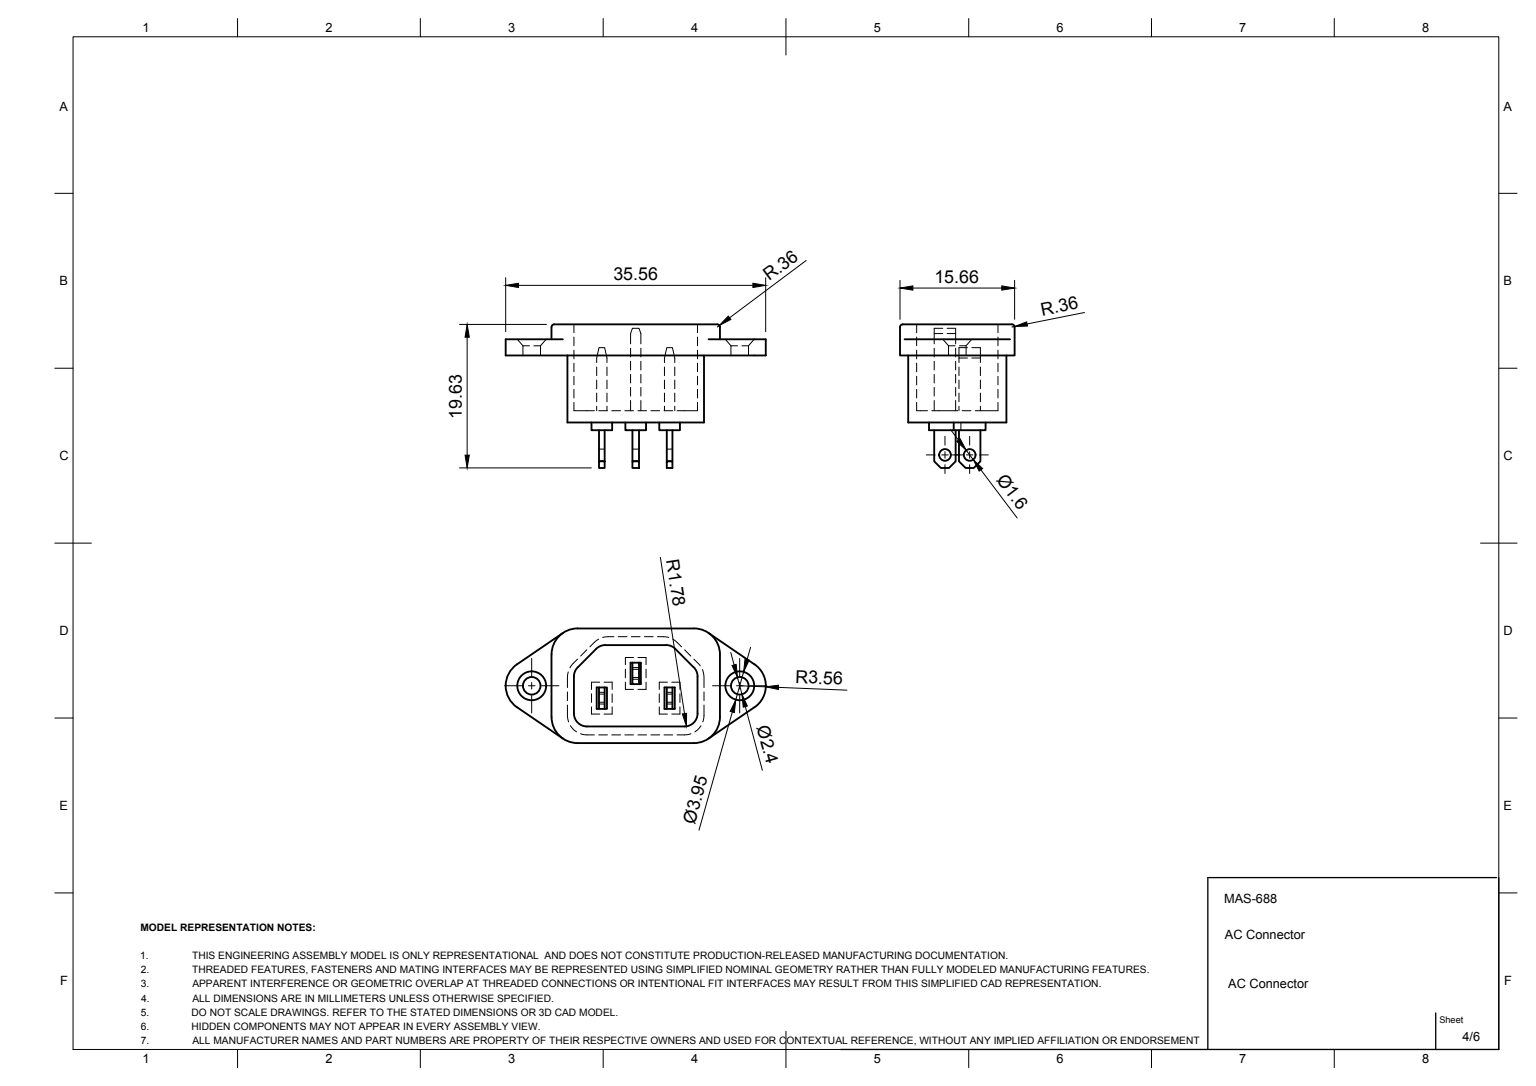
ISO-10303-21;
HEADER;
/* Generated by software containing ST-Developer
 * from STEP Tools, Inc. (www.steptools.com) 
 */

FILE_DESCRIPTION(
/* description */ ('STEP AP214'),
/* implementation_level */ '2;1');

FILE_NAME(
/* name */ 'AC Connector.step',
/* time_stamp */ '2026-11-14T03:58:36-08:00',
/* author */ (''),
/* organization */ (''),
/* preprocessor_version */ 'ST-DEVELOPER v20.2',
/* originating_system */ 'Autodesk Translation Framework v15.17.0.0',
/* authorisation */ '');

FILE_SCHEMA (('AUTOMOTIVE_DESIGN { 1 0 10303 214 3 1 1 }'));
ENDSEC;

DATA;
#10=MECHANICAL_DESIGN_GEOMETRIC_PRESENTATION_REPRESENTATION('',(#42),#65304);
#31=CONICAL_SURFACE('',#41051,1.97294590991864,0.71558499331768);
#32=CONICAL_SURFACE('',#41055,1.97294590991864,0.71558499331768);
#34=SHAPE_REPRESENTATION_RELATIONSHIP('SRR','None',#65325,#38);
#38=ADVANCED_BREP_SHAPE_REPRESENTATION('',(#46),#65301);
#42=STYLED_ITEM('',(#65354),#46);
#46=MANIFOLD_SOLID_BREP('Body1',#39934);
#226=FACE_BOUND('',#4996,.T.);
#227=FACE_BOUND('',#4997,.T.);
#228=FACE_BOUND('',#4998,.T.);
#229=FACE_BOUND('',#5012,.T.);
#230=FACE_BOUND('',#5013,.T.);
#231=FACE_BOUND('',#5014,.T.);
#232=FACE_BOUND('',#5016,.T.);
#233=FACE_BOUND('',#5018,.T.);
#234=FACE_BOUND('',#5019,.T.);
#235=FACE_BOUND('',#5020,.T.);
#236=FACE_BOUND('',#5033,.T.);
#237=FACE_BOUND('',#5037,.T.);
#238=FACE_BOUND('',#5080,.T.);
#239=FACE_BOUND('',#5090,.T.);
#240=FACE_BOUND('',#5093,.T.);
#241=FACE_BOUND('',#5099,.T.);
#242=FACE_BOUND('',#5106,.T.);
#243=FACE_BOUND('',#5108,.T.);
#244=FACE_BOUND('',#5110,.T.);
#245=FACE_BOUND('',#5121,.T.);
#246=FACE_BOUND('',#5123,.T.);
#887=PLANE('',#41066);
#888=PLANE('',#41073);
#889=PLANE('',#41074);
#890=PLANE('',#41075);
#891=PLANE('',#41076);
#892=PLANE('',#41077);
#893=PLANE('',#41078);
#894=PLANE('',#41079);
#895=PLANE('',#41080);
#896=PLANE('',#41081);
#897=PLANE('',#41082);
#898=PLANE('',#41083);
#899=PLANE('',#41084);
#900=PLANE('',#41085);
#901=PLANE('',#41092);
#902=PLANE('',#41103);
#903=PLANE('',#41118);
#904=PLANE('',#41122);
#905=PLANE('',#41126);
#906=PLANE('',#41130);
#907=PLANE('',#41131);
#908=PLANE('',#41134);
#909=PLANE('',#41135);
#910=PLANE('',#41136);
#911=PLANE('',#41137);
#912=PLANE('',#41138);
#913=PLANE('',#41156);
#914=PLANE('',#41158);
#915=PLANE('',#41160);
#916=PLANE('',#41162);
#917=PLANE('',#41164);
#918=PLANE('',#41166);
#919=PLANE('',#41168);
#920=PLANE('',#41170);
#921=PLANE('',#41172);
#922=PLANE('',#41174);
#923=PLANE('',#41176);
#924=PLANE('',#41178);
#925=PLANE('',#41179);
#926=PLANE('',#41180);
#927=PLANE('',#41181);
#928=PLANE('',#41182);
#929=PLANE('',#41183);
#930=PLANE('',#41184);
#931=PLANE('',#41185);
#932=PLANE('',#41186);
#933=PLANE('',#41187);
#934=PLANE('',#41188);
#935=PLANE('',#41189);
#936=PLANE('',#41190);
#937=PLANE('',#41191);
#938=PLANE('',#41192);
#939=PLANE('',#41193);
#940=PLANE('',#41194);
#941=PLANE('',#41195);
#942=PLANE('',#41196);
#943=PLANE('',#41197);
#944=PLANE('',#41198);
#945=PLANE('',#41199);
#946=PLANE('',#41200);
#947=PLANE('',#41201);
#948=PLANE('',#41202);
#949=PLANE('',#41203);
#950=PLANE('',#41204);
#951=PLANE('',#41205);
#952=PLANE('',#41206);
#953=PLANE('',#41207);
#954=PLANE('',#41208);
#955=PLANE('',#41209);
#956=PLANE('',#41210);
#957=PLANE('',#41211);
#958=PLANE('',#41212);
#959=PLANE('',#41213);
#960=PLANE('',#41214);
#961=PLANE('',#41215);
#962=PLANE('',#41216);
#963=PLANE('',#41217);
#964=PLANE('',#41218);
#965=PLANE('',#41219);
#966=PLANE('',#41220);
#967=PLANE('',#41221);
#968=PLANE('',#41222);
#969=PLANE('',#41223);
#2185=TOROIDAL_SURFACE('',#41139,3.2004,0.3556);
#2186=TOROIDAL_SURFACE('',#41146,3.2004,0.3556);
#2187=TOROIDAL_SURFACE('',#41148,3.2004,0.3556);
#2188=TOROIDAL_SURFACE('',#41154,3.2004,0.3556);
#2895=FACE_OUTER_BOUND('',#4987,.T.);
#2896=FACE_OUTER_BOUND('',#4988,.T.);
#2897=FACE_OUTER_BOUND('',#4989,.T.);
#2898=FACE_OUTER_BOUND('',#4990,.T.);
#2899=FACE_OUTER_BOUND('',#4991,.T.);
#2900=FACE_OUTER_BOUND('',#4992,.T.);
#2901=FACE_OUTER_BOUND('',#4993,.T.);
#2902=FACE_OUTER_BOUND('',#4994,.T.);
#2903=FACE_OUTER_BOUND('',#4995,.T.);
#2904=FACE_OUTER_BOUND('',#4999,.T.);
#2905=FACE_OUTER_BOUND('',#5000,.T.);
#2906=FACE_OUTER_BOUND('',#5001,.T.);
#2907=FACE_OUTER_BOUND('',#5002,.T.);
#2908=FACE_OUTER_BOUND('',#5003,.T.);
#2909=FACE_OUTER_BOUND('',#5004,.T.);
#2910=FACE_OUTER_BOUND('',#5005,.T.);
#2911=FACE_OUTER_BOUND('',#5006,.T.);
#2912=FACE_OUTER_BOUND('',#5007,.T.);
#2913=FACE_OUTER_BOUND('',#5008,.T.);
#2914=FACE_OUTER_BOUND('',#5009,.T.);
#2915=FACE_OUTER_BOUND('',#5010,.T.);
#2916=FACE_OUTER_BOUND('',#5011,.T.);
#2917=FACE_OUTER_BOUND('',#5015,.T.);
#2918=FACE_OUTER_BOUND('',#5017,.T.);
#2919=FACE_OUTER_BOUND('',#5021,.T.);
#2920=FACE_OUTER_BOUND('',#5022,.T.);
#2921=FACE_OUTER_BOUND('',#5023,.T.);
#2922=FACE_OUTER_BOUND('',#5024,.T.);
#2923=FACE_OUTER_BOUND('',#5025,.T.);
#2924=FACE_OUTER_BOUND('',#5026,.T.);
#2925=FACE_OUTER_BOUND('',#5027,.T.);
#2926=FACE_OUTER_BOUND('',#5028,.T.);
#2927=FACE_OUTER_BOUND('',#5029,.T.);
#2928=FACE_OUTER_BOUND('',#5030,.T.);
#2929=FACE_OUTER_BOUND('',#5031,.T.);
#2930=FACE_OUTER_BOUND('',#5032,.T.);
#2931=FACE_OUTER_BOUND('',#5034,.T.);
#2932=FACE_OUTER_BOUND('',#5035,.T.);
#2933=FACE_OUTER_BOUND('',#5036,.T.);
#2934=FACE_OUTER_BOUND('',#5038,.T.);
#2935=FACE_OUTER_BOUND('',#5039,.T.);
#2936=FACE_OUTER_BOUND('',#5040,.T.);
#2937=FACE_OUTER_BOUND('',#5041,.T.);
#2938=FACE_OUTER_BOUND('',#5042,.T.);
#2939=FACE_OUTER_BOUND('',#5043,.T.);
#2940=FACE_OUTER_BOUND('',#5044,.T.);
#2941=FACE_OUTER_BOUND('',#5045,.T.);
#2942=FACE_OUTER_BOUND('',#5046,.T.);
#2943=FACE_OUTER_BOUND('',#5047,.T.);
#2944=FACE_OUTER_BOUND('',#5048,.T.);
#2945=FACE_OUTER_BOUND('',#5049,.T.);
#2946=FACE_OUTER_BOUND('',#5050,.T.);
#2947=FACE_OUTER_BOUND('',#5051,.T.);
#2948=FACE_OUTER_BOUND('',#5052,.T.);
#2949=FACE_OUTER_BOUND('',#5053,.T.);
#2950=FACE_OUTER_BOUND('',#5054,.T.);
#2951=FACE_OUTER_BOUND('',#5055,.T.);
#2952=FACE_OUTER_BOUND('',#5056,.T.);
#2953=FACE_OUTER_BOUND('',#5057,.T.);
#2954=FACE_OUTER_BOUND('',#5058,.T.);
#2955=FACE_OUTER_BOUND('',#5059,.T.);
#2956=FACE_OUTER_BOUND('',#5060,.T.);
#2957=FACE_OUTER_BOUND('',#5061,.T.);
#2958=FACE_OUTER_BOUND('',#5062,.T.);
#2959=FACE_OUTER_BOUND('',#5063,.T.);
#2960=FACE_OUTER_BOUND('',#5064,.T.);
#2961=FACE_OUTER_BOUND('',#5065,.T.);
#2962=FACE_OUTER_BOUND('',#5066,.T.);
#2963=FACE_OUTER_BOUND('',#5067,.T.);
#2964=FACE_OUTER_BOUND('',#5068,.T.);
#2965=FACE_OUTER_BOUND('',#5069,.T.);
#2966=FACE_OUTER_BOUND('',#5070,.T.);
#2967=FACE_OUTER_BOUND('',#5071,.T.);
#2968=FACE_OUTER_BOUND('',#5072,.T.);
#2969=FACE_OUTER_BOUND('',#5073,.T.);
#2970=FACE_OUTER_BOUND('',#5074,.T.);
#2971=FACE_OUTER_BOUND('',#5075,.T.);
#2972=FACE_OUTER_BOUND('',#5076,.T.);
#2973=FACE_OUTER_BOUND('',#5077,.T.);
#2974=FACE_OUTER_BOUND('',#5078,.T.);
#2975=FACE_OUTER_BOUND('',#5079,.T.);
#2976=FACE_OUTER_BOUND('',#5081,.T.);
#2977=FACE_OUTER_BOUND('',#5082,.T.);
#2978=FACE_OUTER_BOUND('',#5083,.T.);
#2979=FACE_OUTER_BOUND('',#5084,.T.);
#2980=FACE_OUTER_BOUND('',#5085,.T.);
#2981=FACE_OUTER_BOUND('',#5086,.T.);
#2982=FACE_OUTER_BOUND('',#5087,.T.);
#2983=FACE_OUTER_BOUND('',#5088,.T.);
#2984=FACE_OUTER_BOUND('',#5089,.T.);
#2985=FACE_OUTER_BOUND('',#5091,.T.);
#2986=FACE_OUTER_BOUND('',#5092,.T.);
#2987=FACE_OUTER_BOUND('',#5094,.T.);
#2988=FACE_OUTER_BOUND('',#5095,.T.);
#2989=FACE_OUTER_BOUND('',#5096,.T.);
#2990=FACE_OUTER_BOUND('',#5097,.T.);
#2991=FACE_OUTER_BOUND('',#5098,.T.);
#2992=FACE_OUTER_BOUND('',#5100,.T.);
#2993=FACE_OUTER_BOUND('',#5101,.T.);
#2994=FACE_OUTER_BOUND('',#5102,.T.);
#2995=FACE_OUTER_BOUND('',#5103,.T.);
#2996=FACE_OUTER_BOUND('',#5104,.T.);
#2997=FACE_OUTER_BOUND('',#5105,.T.);
#2998=FACE_OUTER_BOUND('',#5107,.T.);
#2999=FACE_OUTER_BOUND('',#5109,.T.);
#3000=FACE_OUTER_BOUND('',#5111,.T.);
#3001=FACE_OUTER_BOUND('',#5112,.T.);
#3002=FACE_OUTER_BOUND('',#5113,.T.);
#3003=FACE_OUTER_BOUND('',#5114,.T.);
#3004=FACE_OUTER_BOUND('',#5115,.T.);
#3005=FACE_OUTER_BOUND('',#5116,.T.);
#3006=FACE_OUTER_BOUND('',#5117,.T.);
#3007=FACE_OUTER_BOUND('',#5118,.T.);
#3008=FACE_OUTER_BOUND('',#5119,.T.);
#3009=FACE_OUTER_BOUND('',#5120,.T.);
#3010=FACE_OUTER_BOUND('',#5122,.T.);
#4987=EDGE_LOOP('',(#29809,#29810,#29811,#29812));
#4988=EDGE_LOOP('',(#29813,#29814,#29815,#29816));
#4989=EDGE_LOOP('',(#29817,#29818,#29819,#29820));
#4990=EDGE_LOOP('',(#29821,#29822,#29823,#29824,#29825));
#4991=EDGE_LOOP('',(#29826,#29827,#29828,#29829,#29830));
#4992=EDGE_LOOP('',(#29831,#29832,#29833,#29834,#29835));
#4993=EDGE_LOOP('',(#29836,#29837,#29838,#29839));
#4994=EDGE_LOOP('',(#29840,#29841,#29842,#29843,#29844));
#4995=EDGE_LOOP('',(#29845,#29846,#29847,#29848,#29849,#29850,#29851,#29852,
#29853,#29854,#29855,#29856));
#4996=EDGE_LOOP('',(#29857,#29858,#29859,#29860));
#4997=EDGE_LOOP('',(#29861,#29862,#29863,#29864));
#4998=EDGE_LOOP('',(#29865,#29866,#29867,#29868));
#4999=EDGE_LOOP('',(#29869,#29870,#29871,#29872));
#5000=EDGE_LOOP('',(#29873,#29874,#29875,#29876,#29877,#29878));
#5001=EDGE_LOOP('',(#29879,#29880,#29881,#29882,#29883,#29884));
#5002=EDGE_LOOP('',(#29885,#29886,#29887,#29888));
#5003=EDGE_LOOP('',(#29889,#29890,#29891,#29892,#29893,#29894));
#5004=EDGE_LOOP('',(#29895,#29896,#29897,#29898));
#5005=EDGE_LOOP('',(#29899,#29900,#29901,#29902,#29903,#29904));
#5006=EDGE_LOOP('',(#29905,#29906,#29907,#29908));
#5007=EDGE_LOOP('',(#29909,#29910,#29911,#29912));
#5008=EDGE_LOOP('',(#29913,#29914,#29915,#29916,#29917,#29918));
#5009=EDGE_LOOP('',(#29919,#29920,#29921,#29922,#29923,#29924));
#5010=EDGE_LOOP('',(#29925,#29926,#29927,#29928));
#5011=EDGE_LOOP('',(#29929,#29930,#29931,#29932,#29933,#29934,#29935,#29936,
#29937,#29938,#29939,#29940));
#5012=EDGE_LOOP('',(#29941,#29942,#29943,#29944));
#5013=EDGE_LOOP('',(#29945,#29946,#29947,#29948));
#5014=EDGE_LOOP('',(#29949,#29950,#29951,#29952));
#5015=EDGE_LOOP('',(#29953,#29954,#29955,#29956,#29957,#29958,#29959,#29960));
#5016=EDGE_LOOP('',(#29961,#29962,#29963,#29964,#29965,#29966,#29967,#29968,
#29969,#29970,#29971,#29972));
#5017=EDGE_LOOP('',(#29973,#29974,#29975,#29976,#29977,#29978,#29979,#29980,
#29981,#29982,#29983,#29984));
#5018=EDGE_LOOP('',(#29985));
#5019=EDGE_LOOP('',(#29986));
#5020=EDGE_LOOP('',(#29987,#29988,#29989,#29990,#29991,#29992,#29993,#29994,
#29995,#29996,#29997,#29998));
#5021=EDGE_LOOP('',(#29999,#30000,#30001,#30002,#30003,#30004));
#5022=EDGE_LOOP('',(#30005,#30006,#30007,#30008));
#5023=EDGE_LOOP('',(#30009,#30010,#30011,#30012,#30013,#30014));
#5024=EDGE_LOOP('',(#30015,#30016,#30017,#30018));
#5025=EDGE_LOOP('',(#30019,#30020,#30021,#30022,#30023,#30024));
#5026=EDGE_LOOP('',(#30025,#30026,#30027,#30028));
#5027=EDGE_LOOP('',(#30029,#30030,#30031,#30032,#30033,#30034));
#5028=EDGE_LOOP('',(#30035,#30036,#30037,#30038));
#5029=EDGE_LOOP('',(#30039,#30040,#30041,#30042));
#5030=EDGE_LOOP('',(#30043,#30044,#30045,#30046));
#5031=EDGE_LOOP('',(#30047,#30048,#30049,#30050));
#5032=EDGE_LOOP('',(#30051,#30052,#30053,#30054,#30055,#30056));
#5033=EDGE_LOOP('',(#30057));
#5034=EDGE_LOOP('',(#30058,#30059,#30060,#30061));
#5035=EDGE_LOOP('',(#30062,#30063,#30064,#30065));
#5036=EDGE_LOOP('',(#30066,#30067,#30068,#30069,#30070,#30071));
#5037=EDGE_LOOP('',(#30072));
#5038=EDGE_LOOP('',(#30073,#30074,#30075,#30076));
#5039=EDGE_LOOP('',(#30077,#30078,#30079,#30080));
#5040=EDGE_LOOP('',(#30081,#30082,#30083,#30084));
#5041=EDGE_LOOP('',(#30085,#30086,#30087,#30088));
#5042=EDGE_LOOP('',(#30089,#30090,#30091,#30092));
#5043=EDGE_LOOP('',(#30093,#30094,#30095,#30096));
#5044=EDGE_LOOP('',(#30097,#30098,#30099,#30100));
#5045=EDGE_LOOP('',(#30101,#30102,#30103,#30104));
#5046=EDGE_LOOP('',(#30105,#30106,#30107,#30108));
#5047=EDGE_LOOP('',(#30109,#30110,#30111,#30112));
#5048=EDGE_LOOP('',(#30113,#30114,#30115,#30116));
#5049=EDGE_LOOP('',(#30117,#30118,#30119,#30120));
#5050=EDGE_LOOP('',(#30121,#30122,#30123,#30124));
#5051=EDGE_LOOP('',(#30125,#30126,#30127,#30128));
#5052=EDGE_LOOP('',(#30129,#30130,#30131,#30132));
#5053=EDGE_LOOP('',(#30133,#30134,#30135,#30136));
#5054=EDGE_LOOP('',(#30137,#30138,#30139,#30140));
#5055=EDGE_LOOP('',(#30141,#30142,#30143,#30144));
#5056=EDGE_LOOP('',(#30145,#30146,#30147,#30148));
#5057=EDGE_LOOP('',(#30149,#30150,#30151,#30152));
#5058=EDGE_LOOP('',(#30153,#30154,#30155,#30156));
#5059=EDGE_LOOP('',(#30157,#30158,#30159,#30160));
#5060=EDGE_LOOP('',(#30161,#30162,#30163,#30164));
#5061=EDGE_LOOP('',(#30165,#30166,#30167,#30168));
#5062=EDGE_LOOP('',(#30169,#30170,#30171,#30172));
#5063=EDGE_LOOP('',(#30173,#30174,#30175,#30176));
#5064=EDGE_LOOP('',(#30177,#30178,#30179,#30180));
#5065=EDGE_LOOP('',(#30181,#30182,#30183,#30184));
#5066=EDGE_LOOP('',(#30185,#30186,#30187,#30188));
#5067=EDGE_LOOP('',(#30189,#30190,#30191,#30192));
#5068=EDGE_LOOP('',(#30193,#30194,#30195,#30196));
#5069=EDGE_LOOP('',(#30197,#30198,#30199,#30200));
#5070=EDGE_LOOP('',(#30201,#30202,#30203,#30204));
#5071=EDGE_LOOP('',(#30205,#30206,#30207,#30208));
#5072=EDGE_LOOP('',(#30209,#30210,#30211,#30212));
#5073=EDGE_LOOP('',(#30213,#30214,#30215,#30216));
#5074=EDGE_LOOP('',(#30217,#30218,#30219,#30220));
#5075=EDGE_LOOP('',(#30221,#30222,#30223,#30224));
#5076=EDGE_LOOP('',(#30225,#30226,#30227,#30228));
#5077=EDGE_LOOP('',(#30229,#30230,#30231,#30232));
#5078=EDGE_LOOP('',(#30233,#30234,#30235,#30236));
#5079=EDGE_LOOP('',(#30237,#30238,#30239,#30240));
#5080=EDGE_LOOP('',(#30241,#30242,#30243,#30244));
#5081=EDGE_LOOP('',(#30245,#30246,#30247,#30248));
#5082=EDGE_LOOP('',(#30249,#30250,#30251,#30252));
#5083=EDGE_LOOP('',(#30253,#30254,#30255,#30256));
#5084=EDGE_LOOP('',(#30257,#30258,#30259,#30260));
#5085=EDGE_LOOP('',(#30261,#30262,#30263,#30264));
#5086=EDGE_LOOP('',(#30265,#30266,#30267,#30268));
#5087=EDGE_LOOP('',(#30269,#30270,#30271,#30272));
#5088=EDGE_LOOP('',(#30273,#30274,#30275,#30276));
#5089=EDGE_LOOP('',(#30277,#30278,#30279,#30280,#30281,#30282));
#5090=EDGE_LOOP('',(#30283));
#5091=EDGE_LOOP('',(#30284,#30285,#30286,#30287));
#5092=EDGE_LOOP('',(#30288,#30289,#30290,#30291,#30292,#30293));
#5093=EDGE_LOOP('',(#30294));
#5094=EDGE_LOOP('',(#30295,#30296,#30297,#30298));
#5095=EDGE_LOOP('',(#30299,#30300,#30301,#30302));
#5096=EDGE_LOOP('',(#30303,#30304,#30305,#30306));
#5097=EDGE_LOOP('',(#30307,#30308,#30309,#30310));
#5098=EDGE_LOOP('',(#30311,#30312,#30313,#30314));
#5099=EDGE_LOOP('',(#30315,#30316,#30317,#30318));
#5100=EDGE_LOOP('',(#30319,#30320,#30321,#30322));
#5101=EDGE_LOOP('',(#30323,#30324,#30325,#30326));
#5102=EDGE_LOOP('',(#30327,#30328,#30329,#30330));
#5103=EDGE_LOOP('',(#30331,#30332,#30333,#30334));
#5104=EDGE_LOOP('',(#30335,#30336,#30337,#30338));
#5105=EDGE_LOOP('',(#30339,#30340,#30341,#30342,#30343,#30344));
#5106=EDGE_LOOP('',(#30345));
#5107=EDGE_LOOP('',(#30346,#30347,#30348,#30349,#30350,#30351));
#5108=EDGE_LOOP('',(#30352));
#5109=EDGE_LOOP('',(#30353,#30354,#30355,#30356));
#5110=EDGE_LOOP('',(#30357,#30358,#30359,#30360));
#5111=EDGE_LOOP('',(#30361,#30362,#30363,#30364));
#5112=EDGE_LOOP('',(#30365,#30366,#30367,#30368));
#5113=EDGE_LOOP('',(#30369,#30370,#30371,#30372));
#5114=EDGE_LOOP('',(#30373,#30374,#30375,#30376));
#5115=EDGE_LOOP('',(#30377,#30378,#30379,#30380));
#5116=EDGE_LOOP('',(#30381,#30382,#30383,#30384));
#5117=EDGE_LOOP('',(#30385,#30386,#30387,#30388));
#5118=EDGE_LOOP('',(#30389,#30390,#30391,#30392));
#5119=EDGE_LOOP('',(#30393,#30394,#30395,#30396));
#5120=EDGE_LOOP('',(#30397,#30398,#30399,#30400,#30401,#30402));
#5121=EDGE_LOOP('',(#30403));
#5122=EDGE_LOOP('',(#30404,#30405,#30406,#30407,#30408,#30409));
#5123=EDGE_LOOP('',(#30410));
#7776=LINE('',#57368,#12651);
#7777=LINE('',#57374,#12652);
#7778=LINE('',#57380,#12653);
#7779=LINE('',#57388,#12654);
#7780=LINE('',#57396,#12655);
#7781=LINE('',#57400,#12656);
#7782=LINE('',#57407,#12657);
#7783=LINE('',#57410,#12658);
#7784=LINE('',#57413,#12659);
#7785=LINE('',#57420,#12660);
#7786=LINE('',#57424,#12661);
#7787=LINE('',#57428,#12662);
#7788=LINE('',#57432,#12663);
#7789=LINE('',#57436,#12664);
#7790=LINE('',#57439,#12665);
#7791=LINE('',#57442,#12666);
#7792=LINE('',#57444,#12667);
#7793=LINE('',#57446,#12668);
#7794=LINE('',#57447,#12669);
#7795=LINE('',#57450,#12670);
#7796=LINE('',#57452,#12671);
#7797=LINE('',#57454,#12672);
#7798=LINE('',#57455,#12673);
#7799=LINE('',#57458,#12674);
#7800=LINE('',#57460,#12675);
#7801=LINE('',#57462,#12676);
#7802=LINE('',#57463,#12677);
#7803=LINE('',#57467,#12678);
#7804=LINE('',#57469,#12679);
#7805=LINE('',#57471,#12680);
#7806=LINE('',#57472,#12681);
#7807=LINE('',#57476,#12682);
#7808=LINE('',#57478,#12683);
#7809=LINE('',#57479,#12684);
#7810=LINE('',#57481,#12685);
#7811=LINE('',#57482,#12686);
#7812=LINE('',#57486,#12687);
#7813=LINE('',#57488,#12688);
#7814=LINE('',#57489,#12689);
#7815=LINE('',#57491,#12690);
#7816=LINE('',#57492,#12691);
#7817=LINE('',#57494,#12692);
#7818=LINE('',#57495,#12693);
#7819=LINE('',#57499,#12694);
#7820=LINE('',#57501,#12695);
#7821=LINE('',#57503,#12696);
#7822=LINE('',#57505,#12697);
#7823=LINE('',#57507,#12698);
#7824=LINE('',#57508,#12699);
#7825=LINE('',#57512,#12700);
#7826=LINE('',#57513,#12701);
#7827=LINE('',#57514,#12702);
#7828=LINE('',#57517,#12703);
#7829=LINE('',#57519,#12704);
#7830=LINE('',#57521,#12705);
#7831=LINE('',#57523,#12706);
#7832=LINE('',#57524,#12707);
#7833=LINE('',#57526,#12708);
#7834=LINE('',#57527,#12709);
#7835=LINE('',#57531,#12710);
#7836=LINE('',#57533,#12711);
#7837=LINE('',#57535,#12712);
#7838=LINE('',#57536,#12713);
#7839=LINE('',#57540,#12714);
#7840=LINE('',#57541,#12715);
#7841=LINE('',#57543,#12716);
#7842=LINE('',#57545,#12717);
#7843=LINE('',#57546,#12718);
#7844=LINE('',#57549,#12719);
#7845=LINE('',#57551,#12720);
#7846=LINE('',#57553,#12721);
#7847=LINE('',#57555,#12722);
#7848=LINE('',#57556,#12723);
#7849=LINE('',#57558,#12724);
#7850=LINE('',#57559,#12725);
#7851=LINE('',#57565,#12726);
#7852=LINE('',#57569,#12727);
#7853=LINE('',#57573,#12728);
#7854=LINE('',#57577,#12729);
#7855=LINE('',#57581,#12730);
#7856=LINE('',#57584,#12731);
#7857=LINE('',#57585,#12732);
#7858=LINE('',#57586,#12733);
#7859=LINE('',#57587,#12734);
#7860=LINE('',#57591,#12735);
#7861=LINE('',#57595,#12736);
#7862=LINE('',#57599,#12737);
#7863=LINE('',#57603,#12738);
#7864=LINE('',#57609,#12739);
#7865=LINE('',#57613,#12740);
#7866=LINE('',#57617,#12741);
#7867=LINE('',#57621,#12742);
#7868=LINE('',#57625,#12743);
#7869=LINE('',#57628,#12744);
#7870=LINE('',#57631,#12745);
#7871=LINE('',#57635,#12746);
#7872=LINE('',#57639,#12747);
#7873=LINE('',#57643,#12748);
#7874=LINE('',#57647,#12749);
#7875=LINE('',#57650,#12750);
#7876=LINE('',#57653,#12751);
#7877=LINE('',#57657,#12752);
#7878=LINE('',#57661,#12753);
#7879=LINE('',#57665,#12754);
#7880=LINE('',#57669,#12755);
#7881=LINE('',#57673,#12756);
#7882=LINE('',#57678,#12757);
#7883=LINE('',#57681,#12758);
#7884=LINE('',#57683,#12759);
#7885=LINE('',#57688,#12760);
#7886=LINE('',#57689,#12761);
#7887=LINE('',#57690,#12762);
#7888=LINE('',#57694,#12763);
#7889=LINE('',#57697,#12764);
#7890=LINE('',#57699,#12765);
#7891=LINE('',#57704,#12766);
#7892=LINE('',#57705,#12767);
#7893=LINE('',#57706,#12768);
#7894=LINE('',#57709,#12769);
#7895=LINE('',#57713,#12770);
#7896=LINE('',#57715,#12771);
#7897=LINE('',#57718,#12772);
#7898=LINE('',#57722,#12773);
#7899=LINE('',#57724,#12774);
#7900=LINE('',#57727,#12775);
#7901=LINE('',#57728,#12776);
#7902=LINE('',#57731,#12777);
#7903=LINE('',#57734,#12778);
#7904=LINE('',#57737,#12779);
#7905=LINE('',#57739,#12780);
#7906=LINE('',#57758,#12781);
#7907=LINE('',#57759,#12782);
#7908=LINE('',#57761,#12783);
#7909=LINE('',#57763,#12784);
#7910=LINE('',#57765,#12785);
#7911=LINE('',#57767,#12786);
#7912=LINE('',#57769,#12787);
#7913=LINE('',#57771,#12788);
#7914=LINE('',#57773,#12789);
#7915=LINE('',#57775,#12790);
#7916=LINE('',#57777,#12791);
#7917=LINE('',#57779,#12792);
#7918=LINE('',#57782,#12793);
#7919=LINE('',#57783,#12794);
#7920=LINE('',#57785,#12795);
#7921=LINE('',#57787,#12796);
#7922=LINE('',#57789,#12797);
#7923=LINE('',#57791,#12798);
#7924=LINE('',#57793,#12799);
#7925=LINE('',#57795,#12800);
#7926=LINE('',#57797,#12801);
#7927=LINE('',#57799,#12802);
#7928=LINE('',#57801,#12803);
#7929=LINE('',#57803,#12804);
#7930=LINE('',#57806,#12805);
#7931=LINE('',#57808,#12806);
#7932=LINE('',#57810,#12807);
#7933=LINE('',#57820,#12808);
#7934=LINE('',#57822,#12809);
#7935=LINE('',#57824,#12810);
#7936=LINE('',#57825,#12811);
#7937=LINE('',#57828,#12812);
#7938=LINE('',#57830,#12813);
#7939=LINE('',#57832,#12814);
#7940=LINE('',#57833,#12815);
#7941=LINE('',#57835,#12816);
#7942=LINE('',#57836,#12817);
#7943=LINE('',#57838,#12818);
#7944=LINE('',#57840,#12819);
#7945=LINE('',#57845,#12820);
#7946=LINE('',#57847,#12821);
#7947=LINE('',#57849,#12822);
#7948=LINE('',#57850,#12823);
#7949=LINE('',#57853,#12824);
#7950=LINE('',#57855,#12825);
#7951=LINE('',#57856,#12826);
#7952=LINE('',#57859,#12827);
#7953=LINE('',#57861,#12828);
#7954=LINE('',#57862,#12829);
#7955=LINE('',#57864,#12830);
#7956=LINE('',#57865,#12831);
#7957=LINE('',#57867,#12832);
#7958=LINE('',#57869,#12833);
#7959=LINE('',#57873,#12834);
#7960=LINE('',#57875,#12835);
#7961=LINE('',#57876,#12836);
#7962=LINE('',#57879,#12837);
#7963=LINE('',#57880,#12838);
#7964=LINE('',#57883,#12839);
#7965=LINE('',#57884,#12840);
#7966=LINE('',#57886,#12841);
#7967=LINE('',#57890,#12842);
#7968=LINE('',#57892,#12843);
#7969=LINE('',#57894,#12844);
#7970=LINE('',#57895,#12845);
#7971=LINE('',#57899,#12846);
#7972=LINE('',#57901,#12847);
#7973=LINE('',#57903,#12848);
#7974=LINE('',#57904,#12849);
#7975=LINE('',#57907,#12850);
#7976=LINE('',#57909,#12851);
#7977=LINE('',#57910,#12852);
#7978=LINE('',#57914,#12853);
#7979=LINE('',#57915,#12854);
#7980=LINE('',#57916,#12855);
#7981=LINE('',#57918,#12856);
#7982=LINE('',#57919,#12857);
#7983=LINE('',#57921,#12858);
#7984=LINE('',#57922,#12859);
#7985=LINE('',#57928,#12860);
#7986=LINE('',#57930,#12861);
#7987=LINE('',#57932,#12862);
#7988=LINE('',#57933,#12863);
#7989=LINE('',#57936,#12864);
#7990=LINE('',#57938,#12865);
#7991=LINE('',#57940,#12866);
#7992=LINE('',#57941,#12867);
#7993=LINE('',#57943,#12868);
#7994=LINE('',#57944,#12869);
#7995=LINE('',#57946,#12870);
#7996=LINE('',#57948,#12871);
#7997=LINE('',#57953,#12872);
#7998=LINE('',#57955,#12873);
#7999=LINE('',#57957,#12874);
#8000=LINE('',#57958,#12875);
#8001=LINE('',#57962,#12876);
#8002=LINE('',#57963,#12877);
#8003=LINE('',#57964,#12878);
#8004=LINE('',#57967,#12879);
#8005=LINE('',#57969,#12880);
#8006=LINE('',#57970,#12881);
#8007=LINE('',#57972,#12882);
#8008=LINE('',#57973,#12883);
#8009=LINE('',#57975,#12884);
#8010=LINE('',#57976,#12885);
#12651=VECTOR('',#45672,0.800100000000001);
#12652=VECTOR('',#45679,0.800100000000001);
#12653=VECTOR('',#45686,0.800100000000001);
#12654=VECTOR('',#45695,1.97294590991864);
#12655=VECTOR('',#45704,1.97294590991864);
#12656=VECTOR('',#45709,1.20015);
#12657=VECTOR('',#45716,1000.);
#12658=VECTOR('',#45719,1000.);
#12659=VECTOR('',#45722,1.20015);
#12660=VECTOR('',#45729,1000.);
#12661=VECTOR('',#45732,1000.);
#12662=VECTOR('',#45735,1000.);
#12663=VECTOR('',#45738,1000.);
#12664=VECTOR('',#45741,1000.);
#12665=VECTOR('',#45744,1000.);
#12666=VECTOR('',#45745,1000.);
#12667=VECTOR('',#45746,1000.);
#12668=VECTOR('',#45747,1000.);
#12669=VECTOR('',#45748,1000.);
#12670=VECTOR('',#45749,1000.);
#12671=VECTOR('',#45750,1000.);
#12672=VECTOR('',#45751,1000.);
#12673=VECTOR('',#45752,1000.);
#12674=VECTOR('',#45753,1000.);
#12675=VECTOR('',#45754,1000.);
#12676=VECTOR('',#45755,1000.);
#12677=VECTOR('',#45756,1000.);
#12678=VECTOR('',#45759,1000.);
#12679=VECTOR('',#45760,1000.);
#12680=VECTOR('',#45761,1000.);
#12681=VECTOR('',#45762,1000.);
#12682=VECTOR('',#45765,1000.);
#12683=VECTOR('',#45766,1000.);
#12684=VECTOR('',#45767,1000.);
#12685=VECTOR('',#45768,1000.);
#12686=VECTOR('',#45769,1000.);
#12687=VECTOR('',#45772,1000.);
#12688=VECTOR('',#45773,1000.);
#12689=VECTOR('',#45774,1000.);
#12690=VECTOR('',#45775,1000.);
#12691=VECTOR('',#45776,1000.);
#12692=VECTOR('',#45779,1000.);
#12693=VECTOR('',#45780,1000.);
#12694=VECTOR('',#45783,1000.);
#12695=VECTOR('',#45784,1000.);
#12696=VECTOR('',#45785,1000.);
#12697=VECTOR('',#45786,1000.);
#12698=VECTOR('',#45787,1000.);
#12699=VECTOR('',#45788,1000.);
#12700=VECTOR('',#45791,1000.);
#12701=VECTOR('',#45792,1000.);
#12702=VECTOR('',#45793,1000.);
#12703=VECTOR('',#45796,1000.);
#12704=VECTOR('',#45797,1000.);
#12705=VECTOR('',#45798,1000.);
#12706=VECTOR('',#45799,1000.);
#12707=VECTOR('',#45800,1000.);
#12708=VECTOR('',#45803,1000.);
#12709=VECTOR('',#45804,1000.);
#12710=VECTOR('',#45807,1000.);
#12711=VECTOR('',#45808,1000.);
#12712=VECTOR('',#45809,1000.);
#12713=VECTOR('',#45810,1000.);
#12714=VECTOR('',#45813,1000.);
#12715=VECTOR('',#45814,1000.);
#12716=VECTOR('',#45815,1000.);
#12717=VECTOR('',#45816,1000.);
#12718=VECTOR('',#45817,1000.);
#12719=VECTOR('',#45820,1000.);
#12720=VECTOR('',#45821,1000.);
#12721=VECTOR('',#45822,1000.);
#12722=VECTOR('',#45823,1000.);
#12723=VECTOR('',#45824,1000.);
#12724=VECTOR('',#45827,1000.);
#12725=VECTOR('',#45828,1000.);
#12726=VECTOR('',#45833,1000.);
#12727=VECTOR('',#45836,1000.);
#12728=VECTOR('',#45839,1000.);
#12729=VECTOR('',#45842,1000.);
#12730=VECTOR('',#45845,1000.);
#12731=VECTOR('',#45848,1000.);
#12732=VECTOR('',#45849,1000.);
#12733=VECTOR('',#45850,1000.);
#12734=VECTOR('',#45851,1000.);
#12735=VECTOR('',#45854,1000.);
#12736=VECTOR('',#45857,1000.);
#12737=VECTOR('',#45860,1000.);
#12738=VECTOR('',#45863,1000.);
#12739=VECTOR('',#45868,1000.);
#12740=VECTOR('',#45871,1000.);
#12741=VECTOR('',#45874,1000.);
#12742=VECTOR('',#45877,1000.);
#12743=VECTOR('',#45880,1000.);
#12744=VECTOR('',#45883,1000.);
#12745=VECTOR('',#45886,1000.);
#12746=VECTOR('',#45889,1000.);
#12747=VECTOR('',#45892,1000.);
#12748=VECTOR('',#45895,1000.);
#12749=VECTOR('',#45898,1000.);
#12750=VECTOR('',#45901,1000.);
#12751=VECTOR('',#45902,1000.);
#12752=VECTOR('',#45905,1000.);
#12753=VECTOR('',#45908,1000.);
#12754=VECTOR('',#45911,1000.);
#12755=VECTOR('',#45914,1000.);
#12756=VECTOR('',#45917,1000.);
#12757=VECTOR('',#45922,1000.);
#12758=VECTOR('',#45925,1000.);
#12759=VECTOR('',#45926,1000.);
#12760=VECTOR('',#45931,1000.);
#12761=VECTOR('',#45932,1000.);
#12762=VECTOR('',#45933,1000.);
#12763=VECTOR('',#45936,1000.);
#12764=VECTOR('',#45939,1000.);
#12765=VECTOR('',#45940,1000.);
#12766=VECTOR('',#45945,1000.);
#12767=VECTOR('',#45946,1000.);
#12768=VECTOR('',#45947,1000.);
#12769=VECTOR('',#45950,1000.);
#12770=VECTOR('',#45955,1000.);
#12771=VECTOR('',#45958,1000.);
#12772=VECTOR('',#45961,1000.);
#12773=VECTOR('',#45966,1000.);
#12774=VECTOR('',#45969,1000.);
#12775=VECTOR('',#45972,1000.);
#12776=VECTOR('',#45973,1000.);
#12777=VECTOR('',#45976,1000.);
#12778=VECTOR('',#45981,1000.);
#12779=VECTOR('',#45986,1000.);
#12780=VECTOR('',#45989,1000.);
#12781=VECTOR('',#46026,1000.);
#12782=VECTOR('',#46027,1000.);
#12783=VECTOR('',#46030,1000.);
#12784=VECTOR('',#46033,1000.);
#12785=VECTOR('',#46036,1000.);
#12786=VECTOR('',#46039,1000.);
#12787=VECTOR('',#46042,1000.);
#12788=VECTOR('',#46045,1000.);
#12789=VECTOR('',#46048,1000.);
#12790=VECTOR('',#46051,1000.);
#12791=VECTOR('',#46054,1000.);
#12792=VECTOR('',#46057,1000.);
#12793=VECTOR('',#46062,1000.);
#12794=VECTOR('',#46063,1000.);
#12795=VECTOR('',#46066,1000.);
#12796=VECTOR('',#46069,1000.);
#12797=VECTOR('',#46072,1000.);
#12798=VECTOR('',#46075,1000.);
#12799=VECTOR('',#46078,1000.);
#12800=VECTOR('',#46081,1000.);
#12801=VECTOR('',#46084,1000.);
#12802=VECTOR('',#46087,1000.);
#12803=VECTOR('',#46090,1000.);
#12804=VECTOR('',#46093,1000.);
#12805=VECTOR('',#46098,1000.);
#12806=VECTOR('',#46101,1000.);
#12807=VECTOR('',#46104,1000.);
#12808=VECTOR('',#46119,1000.);
#12809=VECTOR('',#46120,1000.);
#12810=VECTOR('',#46121,1000.);
#12811=VECTOR('',#46122,1000.);
#12812=VECTOR('',#46123,1000.);
#12813=VECTOR('',#46124,1000.);
#12814=VECTOR('',#46125,1000.);
#12815=VECTOR('',#46126,1000.);
#12816=VECTOR('',#46129,1000.);
#12817=VECTOR('',#46130,1000.);
#12818=VECTOR('',#46133,1000.);
#12819=VECTOR('',#46136,1000.);
#12820=VECTOR('',#46141,1000.);
#12821=VECTOR('',#46142,1000.);
#12822=VECTOR('',#46143,1000.);
#12823=VECTOR('',#46144,1000.);
#12824=VECTOR('',#46147,1000.);
#12825=VECTOR('',#46148,1000.);
#12826=VECTOR('',#46149,1000.);
#12827=VECTOR('',#46152,1000.);
#12828=VECTOR('',#46153,1000.);
#12829=VECTOR('',#46154,1000.);
#12830=VECTOR('',#46157,1000.);
#12831=VECTOR('',#46158,1000.);
#12832=VECTOR('',#46161,1000.);
#12833=VECTOR('',#46164,1000.);
#12834=VECTOR('',#46169,1000.);
#12835=VECTOR('',#46170,1000.);
#12836=VECTOR('',#46171,1000.);
#12837=VECTOR('',#46174,1000.);
#12838=VECTOR('',#46175,1000.);
#12839=VECTOR('',#46178,1000.);
#12840=VECTOR('',#46179,1000.);
#12841=VECTOR('',#46182,1000.);
#12842=VECTOR('',#46185,1000.);
#12843=VECTOR('',#46186,1000.);
#12844=VECTOR('',#46187,1000.);
#12845=VECTOR('',#46188,1000.);
#12846=VECTOR('',#46191,1000.);
#12847=VECTOR('',#46192,1000.);
#12848=VECTOR('',#46193,1000.);
#12849=VECTOR('',#46194,1000.);
#12850=VECTOR('',#46197,1000.);
#12851=VECTOR('',#46198,1000.);
#12852=VECTOR('',#46199,1000.);
#12853=VECTOR('',#46202,1000.);
#12854=VECTOR('',#46203,1000.);
#12855=VECTOR('',#46204,1000.);
#12856=VECTOR('',#46207,1000.);
#12857=VECTOR('',#46208,1000.);
#12858=VECTOR('',#46211,1000.);
#12859=VECTOR('',#46212,1000.);
#12860=VECTOR('',#46219,1000.);
#12861=VECTOR('',#46220,1000.);
#12862=VECTOR('',#46221,1000.);
#12863=VECTOR('',#46222,1000.);
#12864=VECTOR('',#46223,1000.);
#12865=VECTOR('',#46224,1000.);
#12866=VECTOR('',#46225,1000.);
#12867=VECTOR('',#46226,1000.);
#12868=VECTOR('',#46229,1000.);
#12869=VECTOR('',#46230,1000.);
#12870=VECTOR('',#46233,1000.);
#12871=VECTOR('',#46236,1000.);
#12872=VECTOR('',#46241,1000.);
#12873=VECTOR('',#46242,1000.);
#12874=VECTOR('',#46243,1000.);
#12875=VECTOR('',#46244,1000.);
#12876=VECTOR('',#46247,1000.);
#12877=VECTOR('',#46248,1000.);
#12878=VECTOR('',#46249,1000.);
#12879=VECTOR('',#46252,1000.);
#12880=VECTOR('',#46253,1000.);
#12881=VECTOR('',#46254,1000.);
#12882=VECTOR('',#46257,1000.);
#12883=VECTOR('',#46258,1000.);
#12884=VECTOR('',#46261,1000.);
#12885=VECTOR('',#46262,1000.);
#17028=CIRCLE('',#41043,0.800100000000001);
#17029=CIRCLE('',#41044,0.800100000000001);
#17030=CIRCLE('',#41046,0.800100000000001);
#17031=CIRCLE('',#41047,0.800100000000001);
#17032=CIRCLE('',#41049,0.800100000000001);
#17033=CIRCLE('',#41050,0.800100000000001);
#17034=CIRCLE('',#41052,1.20015);
#17035=CIRCLE('',#41053,1.20015);
#17036=CIRCLE('',#41054,1.97294590991864);
#17037=CIRCLE('',#41056,1.20015);
#17038=CIRCLE('',#41057,1.20015);
#17039=CIRCLE('',#41058,1.97294590991864);
#17040=CIRCLE('',#41060,1.20015);
#17041=CIRCLE('',#41062,3.556);
#17042=CIRCLE('',#41063,3.556);
#17043=CIRCLE('',#41065,1.20015);
#17044=CIRCLE('',#41067,2.667);
#17045=CIRCLE('',#41068,2.667);
#17046=CIRCLE('',#41069,2.667);
#17047=CIRCLE('',#41070,2.66700000000001);
#17048=CIRCLE('',#41071,2.667);
#17049=CIRCLE('',#41072,2.667);
#17050=CIRCLE('',#41086,1.778);
#17051=CIRCLE('',#41087,1.778);
#17052=CIRCLE('',#41088,1.778);
#17053=CIRCLE('',#41089,1.778);
#17054=CIRCLE('',#41090,1.778);
#17055=CIRCLE('',#41091,1.778);
#17056=CIRCLE('',#41093,3.2004);
#17057=CIRCLE('',#41094,3.2004);
#17058=CIRCLE('',#41095,3.2004);
#17059=CIRCLE('',#41096,3.2004);
#17060=CIRCLE('',#41097,1.778);
#17061=CIRCLE('',#41098,1.778);
#17062=CIRCLE('',#41099,1.778);
#17063=CIRCLE('',#41100,1.778);
#17064=CIRCLE('',#41101,1.778);
#17065=CIRCLE('',#41102,1.778);
#17066=CIRCLE('',#41104,3.556);
#17067=CIRCLE('',#41105,3.556);
#17068=CIRCLE('',#41106,3.556);
#17069=CIRCLE('',#41107,3.556);
#17070=CIRCLE('',#41108,3.556);
#17071=CIRCLE('',#41109,2.667);
#17072=CIRCLE('',#41110,2.667);
#17073=CIRCLE('',#41111,2.667);
#17074=CIRCLE('',#41112,2.66700000000001);
#17075=CIRCLE('',#41113,2.667);
#17076=CIRCLE('',#41114,2.667);
#17077=CIRCLE('',#41116,3.556);
#17078=CIRCLE('',#41117,3.556);
#17079=CIRCLE('',#41120,3.556);
#17080=CIRCLE('',#41121,3.556);
#17081=CIRCLE('',#41124,3.556);
#17082=CIRCLE('',#41125,3.556);
#17083=CIRCLE('',#41128,3.556);
#17084=CIRCLE('',#41129,3.556);
#17085=CIRCLE('',#41133,3.556);
#17086=CIRCLE('',#41140,0.3556);
#17087=CIRCLE('',#41141,0.3556);
#17088=CIRCLE('',#41143,0.3556);
#17089=CIRCLE('',#41145,0.3556);
#17090=CIRCLE('',#41147,0.3556);
#17091=CIRCLE('',#41149,0.3556);
#17092=CIRCLE('',#41151,0.3556);
#17093=CIRCLE('',#41153,0.355599999999999);
#18238=VERTEX_POINT('',#57365);
#18239=VERTEX_POINT('',#57367);
#18240=VERTEX_POINT('',#57371);
#18241=VERTEX_POINT('',#57373);
#18242=VERTEX_POINT('',#57377);
#18243=VERTEX_POINT('',#57379);
#18244=VERTEX_POINT('',#57383);
#18245=VERTEX_POINT('',#57384);
#18246=VERTEX_POINT('',#57387);
#18247=VERTEX_POINT('',#57391);
#18248=VERTEX_POINT('',#57392);
#18249=VERTEX_POINT('',#57395);
#18250=VERTEX_POINT('',#57399);
#18251=VERTEX_POINT('',#57403);
#18252=VERTEX_POINT('',#57404);
#18253=VERTEX_POINT('',#57406);
#18254=VERTEX_POINT('',#57408);
#18255=VERTEX_POINT('',#57412);
#18256=VERTEX_POINT('',#57416);
#18257=VERTEX_POINT('',#57417);
#18258=VERTEX_POINT('',#57419);
#18259=VERTEX_POINT('',#57421);
#18260=VERTEX_POINT('',#57423);
#18261=VERTEX_POINT('',#57425);
#18262=VERTEX_POINT('',#57427);
#18263=VERTEX_POINT('',#57429);
#18264=VERTEX_POINT('',#57431);
#18265=VERTEX_POINT('',#57433);
#18266=VERTEX_POINT('',#57435);
#18267=VERTEX_POINT('',#57437);
#18268=VERTEX_POINT('',#57440);
#18269=VERTEX_POINT('',#57441);
#18270=VERTEX_POINT('',#57443);
#18271=VERTEX_POINT('',#57445);
#18272=VERTEX_POINT('',#57448);
#18273=VERTEX_POINT('',#57449);
#18274=VERTEX_POINT('',#57451);
#18275=VERTEX_POINT('',#57453);
#18276=VERTEX_POINT('',#57456);
#18277=VERTEX_POINT('',#57457);
#18278=VERTEX_POINT('',#57459);
#18279=VERTEX_POINT('',#57461);
#18280=VERTEX_POINT('',#57465);
#18281=VERTEX_POINT('',#57466);
#18282=VERTEX_POINT('',#57468);
#18283=VERTEX_POINT('',#57470);
#18284=VERTEX_POINT('',#57474);
#18285=VERTEX_POINT('',#57475);
#18286=VERTEX_POINT('',#57477);
#18287=VERTEX_POINT('',#57480);
#18288=VERTEX_POINT('',#57484);
#18289=VERTEX_POINT('',#57485);
#18290=VERTEX_POINT('',#57487);
#18291=VERTEX_POINT('',#57490);
#18292=VERTEX_POINT('',#57497);
#18293=VERTEX_POINT('',#57498);
#18294=VERTEX_POINT('',#57500);
#18295=VERTEX_POINT('',#57502);
#18296=VERTEX_POINT('',#57504);
#18297=VERTEX_POINT('',#57506);
#18298=VERTEX_POINT('',#57510);
#18299=VERTEX_POINT('',#57511);
#18300=VERTEX_POINT('',#57516);
#18301=VERTEX_POINT('',#57518);
#18302=VERTEX_POINT('',#57520);
#18303=VERTEX_POINT('',#57522);
#18304=VERTEX_POINT('',#57529);
#18305=VERTEX_POINT('',#57530);
#18306=VERTEX_POINT('',#57532);
#18307=VERTEX_POINT('',#57534);
#18308=VERTEX_POINT('',#57538);
#18309=VERTEX_POINT('',#57539);
#18310=VERTEX_POINT('',#57542);
#18311=VERTEX_POINT('',#57544);
#18312=VERTEX_POINT('',#57548);
#18313=VERTEX_POINT('',#57550);
#18314=VERTEX_POINT('',#57552);
#18315=VERTEX_POINT('',#57554);
#18316=VERTEX_POINT('',#57561);
#18317=VERTEX_POINT('',#57562);
#18318=VERTEX_POINT('',#57564);
#18319=VERTEX_POINT('',#57566);
#18320=VERTEX_POINT('',#57568);
#18321=VERTEX_POINT('',#57570);
#18322=VERTEX_POINT('',#57572);
#18323=VERTEX_POINT('',#57574);
#18324=VERTEX_POINT('',#57576);
#18325=VERTEX_POINT('',#57578);
#18326=VERTEX_POINT('',#57580);
#18327=VERTEX_POINT('',#57582);
#18328=VERTEX_POINT('',#57589);
#18329=VERTEX_POINT('',#57590);
#18330=VERTEX_POINT('',#57592);
#18331=VERTEX_POINT('',#57594);
#18332=VERTEX_POINT('',#57596);
#18333=VERTEX_POINT('',#57598);
#18334=VERTEX_POINT('',#57600);
#18335=VERTEX_POINT('',#57602);
#18336=VERTEX_POINT('',#57605);
#18337=VERTEX_POINT('',#57606);
#18338=VERTEX_POINT('',#57608);
#18339=VERTEX_POINT('',#57610);
#18340=VERTEX_POINT('',#57612);
#18341=VERTEX_POINT('',#57614);
#18342=VERTEX_POINT('',#57616);
#18343=VERTEX_POINT('',#57618);
#18344=VERTEX_POINT('',#57620);
#18345=VERTEX_POINT('',#57622);
#18346=VERTEX_POINT('',#57624);
#18347=VERTEX_POINT('',#57626);
#18348=VERTEX_POINT('',#57630);
#18349=VERTEX_POINT('',#57632);
#18350=VERTEX_POINT('',#57634);
#18351=VERTEX_POINT('',#57636);
#18352=VERTEX_POINT('',#57638);
#18353=VERTEX_POINT('',#57640);
#18354=VERTEX_POINT('',#57642);
#18355=VERTEX_POINT('',#57644);
#18356=VERTEX_POINT('',#57646);
#18357=VERTEX_POINT('',#57648);
#18358=VERTEX_POINT('',#57651);
#18359=VERTEX_POINT('',#57652);
#18360=VERTEX_POINT('',#57654);
#18361=VERTEX_POINT('',#57656);
#18362=VERTEX_POINT('',#57658);
#18363=VERTEX_POINT('',#57660);
#18364=VERTEX_POINT('',#57662);
#18365=VERTEX_POINT('',#57664);
#18366=VERTEX_POINT('',#57666);
#18367=VERTEX_POINT('',#57668);
#18368=VERTEX_POINT('',#57670);
#18369=VERTEX_POINT('',#57672);
#18370=VERTEX_POINT('',#57676);
#18371=VERTEX_POINT('',#57677);
#18372=VERTEX_POINT('',#57679);
#18373=VERTEX_POINT('',#57682);
#18374=VERTEX_POINT('',#57686);
#18375=VERTEX_POINT('',#57687);
#18376=VERTEX_POINT('',#57692);
#18377=VERTEX_POINT('',#57693);
#18378=VERTEX_POINT('',#57695);
#18379=VERTEX_POINT('',#57698);
#18380=VERTEX_POINT('',#57702);
#18381=VERTEX_POINT('',#57703);
#18382=VERTEX_POINT('',#57708);
#18383=VERTEX_POINT('',#57711);
#18384=VERTEX_POINT('',#57717);
#18385=VERTEX_POINT('',#57720);
#18386=VERTEX_POINT('',#57726);
#18387=VERTEX_POINT('',#57730);
#18388=VERTEX_POINT('',#57818);
#18389=VERTEX_POINT('',#57819);
#18390=VERTEX_POINT('',#57821);
#18391=VERTEX_POINT('',#57823);
#18392=VERTEX_POINT('',#57826);
#18393=VERTEX_POINT('',#57827);
#18394=VERTEX_POINT('',#57829);
#18395=VERTEX_POINT('',#57831);
#18396=VERTEX_POINT('',#57843);
#18397=VERTEX_POINT('',#57844);
#18398=VERTEX_POINT('',#57846);
#18399=VERTEX_POINT('',#57848);
#18400=VERTEX_POINT('',#57852);
#18401=VERTEX_POINT('',#57854);
#18402=VERTEX_POINT('',#57858);
#18403=VERTEX_POINT('',#57860);
#18404=VERTEX_POINT('',#57872);
#18405=VERTEX_POINT('',#57874);
#18406=VERTEX_POINT('',#57878);
#18407=VERTEX_POINT('',#57882);
#18408=VERTEX_POINT('',#57888);
#18409=VERTEX_POINT('',#57889);
#18410=VERTEX_POINT('',#57891);
#18411=VERTEX_POINT('',#57893);
#18412=VERTEX_POINT('',#57897);
#18413=VERTEX_POINT('',#57898);
#18414=VERTEX_POINT('',#57900);
#18415=VERTEX_POINT('',#57902);
#18416=VERTEX_POINT('',#57906);
#18417=VERTEX_POINT('',#57908);
#18418=VERTEX_POINT('',#57912);
#18419=VERTEX_POINT('',#57913);
#18420=VERTEX_POINT('',#57926);
#18421=VERTEX_POINT('',#57927);
#18422=VERTEX_POINT('',#57929);
#18423=VERTEX_POINT('',#57931);
#18424=VERTEX_POINT('',#57934);
#18425=VERTEX_POINT('',#57935);
#18426=VERTEX_POINT('',#57937);
#18427=VERTEX_POINT('',#57939);
#18428=VERTEX_POINT('',#57951);
#18429=VERTEX_POINT('',#57952);
#18430=VERTEX_POINT('',#57954);
#18431=VERTEX_POINT('',#57956);
#18432=VERTEX_POINT('',#57960);
#18433=VERTEX_POINT('',#57961);
#18434=VERTEX_POINT('',#57966);
#18435=VERTEX_POINT('',#57968);
#22522=EDGE_CURVE('',#18238,#18238,#17028,.T.);
#22523=EDGE_CURVE('',#18238,#18239,#7776,.T.);
#22524=EDGE_CURVE('',#18239,#18239,#17029,.T.);
#22525=EDGE_CURVE('',#18240,#18240,#17030,.T.);
#22526=EDGE_CURVE('',#18240,#18241,#7777,.T.);
#22527=EDGE_CURVE('',#18241,#18241,#17031,.T.);
#22528=EDGE_CURVE('',#18242,#18242,#17032,.T.);
#22529=EDGE_CURVE('',#18242,#18243,#7778,.T.);
#22530=EDGE_CURVE('',#18243,#18243,#17033,.T.);
#22531=EDGE_CURVE('',#18244,#18245,#17034,.T.);
#22532=EDGE_CURVE('',#18245,#18244,#17035,.T.);
#22533=EDGE_CURVE('',#18245,#18246,#7779,.T.);
#22534=EDGE_CURVE('',#18246,#18246,#17036,.T.);
#22535=EDGE_CURVE('',#18247,#18248,#17037,.T.);
#22536=EDGE_CURVE('',#18248,#18247,#17038,.T.);
#22537=EDGE_CURVE('',#18248,#18249,#7780,.T.);
#22538=EDGE_CURVE('',#18249,#18249,#17039,.T.);
#22539=EDGE_CURVE('',#18244,#18250,#7781,.T.);
#22540=EDGE_CURVE('',#18250,#18250,#17040,.T.);
#22541=EDGE_CURVE('',#18251,#18252,#17041,.T.);
#22542=EDGE_CURVE('',#18251,#18253,#7782,.T.);
#22543=EDGE_CURVE('',#18253,#18254,#17042,.T.);
#22544=EDGE_CURVE('',#18252,#18254,#7783,.T.);
#22545=EDGE_CURVE('',#18247,#18255,#7784,.T.);
#22546=EDGE_CURVE('',#18255,#18255,#17043,.T.);
#22547=EDGE_CURVE('',#18256,#18257,#17044,.T.);
#22548=EDGE_CURVE('',#18257,#18258,#7785,.T.);
#22549=EDGE_CURVE('',#18259,#18258,#17045,.T.);
#22550=EDGE_CURVE('',#18260,#18259,#7786,.T.);
#22551=EDGE_CURVE('',#18260,#18261,#17046,.T.);
#22552=EDGE_CURVE('',#18261,#18262,#7787,.T.);
#22553=EDGE_CURVE('',#18263,#18262,#17047,.T.);
#22554=EDGE_CURVE('',#18263,#18264,#7788,.T.);
#22555=EDGE_CURVE('',#18264,#18265,#17048,.T.);
#22556=EDGE_CURVE('',#18266,#18265,#7789,.T.);
#22557=EDGE_CURVE('',#18267,#18266,#17049,.T.);
#22558=EDGE_CURVE('',#18256,#18267,#7790,.T.);
#22559=EDGE_CURVE('',#18268,#18269,#7791,.T.);
#22560=EDGE_CURVE('',#18270,#18269,#7792,.T.);
#22561=EDGE_CURVE('',#18270,#18271,#7793,.T.);
#22562=EDGE_CURVE('',#18268,#18271,#7794,.T.);
#22563=EDGE_CURVE('',#18272,#18273,#7795,.T.);
#22564=EDGE_CURVE('',#18274,#18273,#7796,.T.);
#22565=EDGE_CURVE('',#18274,#18275,#7797,.T.);
#22566=EDGE_CURVE('',#18272,#18275,#7798,.T.);
#22567=EDGE_CURVE('',#18276,#18277,#7799,.T.);
#22568=EDGE_CURVE('',#18278,#18277,#7800,.T.);
#22569=EDGE_CURVE('',#18278,#18279,#7801,.T.);
#22570=EDGE_CURVE('',#18276,#18279,#7802,.T.);
#22571=EDGE_CURVE('',#18280,#18281,#7803,.T.);
#22572=EDGE_CURVE('',#18280,#18282,#7804,.T.);
#22573=EDGE_CURVE('',#18282,#18283,#7805,.T.);
#22574=EDGE_CURVE('',#18281,#18283,#7806,.T.);
#22575=EDGE_CURVE('',#18284,#18285,#7807,.T.);
#22576=EDGE_CURVE('',#18284,#18286,#7808,.T.);
#22577=EDGE_CURVE('',#18286,#18281,#7809,.T.);
#22578=EDGE_CURVE('',#18287,#18283,#7810,.T.);
#22579=EDGE_CURVE('',#18285,#18287,#7811,.T.);
#22580=EDGE_CURVE('',#18288,#18289,#7812,.T.);
#22581=EDGE_CURVE('',#18289,#18290,#7813,.T.);
#22582=EDGE_CURVE('',#18282,#18290,#7814,.T.);
#22583=EDGE_CURVE('',#18291,#18280,#7815,.T.);
#22584=EDGE_CURVE('',#18291,#18288,#7816,.T.);
#22585=EDGE_CURVE('',#18284,#18288,#7817,.T.);
#22586=EDGE_CURVE('',#18286,#18291,#7818,.T.);
#22587=EDGE_CURVE('',#18292,#18293,#7819,.T.);
#22588=EDGE_CURVE('',#18294,#18292,#7820,.T.);
#22589=EDGE_CURVE('',#18294,#18295,#7821,.T.);
#22590=EDGE_CURVE('',#18295,#18296,#7822,.T.);
#22591=EDGE_CURVE('',#18296,#18297,#7823,.T.);
#22592=EDGE_CURVE('',#18293,#18297,#7824,.T.);
#22593=EDGE_CURVE('',#18298,#18299,#7825,.T.);
#22594=EDGE_CURVE('',#18298,#18293,#7826,.T.);
#22595=EDGE_CURVE('',#18299,#18297,#7827,.T.);
#22596=EDGE_CURVE('',#18300,#18298,#7828,.T.);
#22597=EDGE_CURVE('',#18299,#18301,#7829,.T.);
#22598=EDGE_CURVE('',#18302,#18301,#7830,.T.);
#22599=EDGE_CURVE('',#18303,#18302,#7831,.T.);
#22600=EDGE_CURVE('',#18300,#18303,#7832,.T.);
#22601=EDGE_CURVE('',#18292,#18300,#7833,.T.);
#22602=EDGE_CURVE('',#18294,#18303,#7834,.T.);
#22603=EDGE_CURVE('',#18304,#18305,#7835,.T.);
#22604=EDGE_CURVE('',#18304,#18306,#7836,.T.);
#22605=EDGE_CURVE('',#18306,#18307,#7837,.T.);
#22606=EDGE_CURVE('',#18305,#18307,#7838,.T.);
#22607=EDGE_CURVE('',#18308,#18309,#7839,.T.);
#22608=EDGE_CURVE('',#18309,#18305,#7840,.T.);
#22609=EDGE_CURVE('',#18310,#18307,#7841,.T.);
#22610=EDGE_CURVE('',#18311,#18310,#7842,.T.);
#22611=EDGE_CURVE('',#18308,#18311,#7843,.T.);
#22612=EDGE_CURVE('',#18304,#18312,#7844,.T.);
#22613=EDGE_CURVE('',#18312,#18313,#7845,.T.);
#22614=EDGE_CURVE('',#18314,#18313,#7846,.T.);
#22615=EDGE_CURVE('',#18314,#18315,#7847,.T.);
#22616=EDGE_CURVE('',#18306,#18315,#7848,.T.);
#22617=EDGE_CURVE('',#18309,#18312,#7849,.T.);
#22618=EDGE_CURVE('',#18308,#18313,#7850,.T.);
#22619=EDGE_CURVE('',#18316,#18317,#17050,.T.);
#22620=EDGE_CURVE('',#18318,#18316,#7851,.T.);
#22621=EDGE_CURVE('',#18318,#18319,#17051,.T.);
#22622=EDGE_CURVE('',#18320,#18319,#7852,.T.);
#22623=EDGE_CURVE('',#18321,#18320,#17052,.T.);
#22624=EDGE_CURVE('',#18321,#18322,#7853,.T.);
#22625=EDGE_CURVE('',#18322,#18323,#17053,.T.);
#22626=EDGE_CURVE('',#18324,#18323,#7854,.T.);
#22627=EDGE_CURVE('',#18325,#18324,#17054,.T.);
#22628=EDGE_CURVE('',#18325,#18326,#7855,.T.);
#22629=EDGE_CURVE('',#18326,#18327,#17055,.T.);
#22630=EDGE_CURVE('',#18327,#18317,#7856,.T.);
#22631=EDGE_CURVE('',#18310,#18315,#7857,.T.);
#22632=EDGE_CURVE('',#18296,#18301,#7858,.T.);
#22633=EDGE_CURVE('',#18287,#18290,#7859,.T.);
#22634=EDGE_CURVE('',#18328,#18329,#7860,.T.);
#22635=EDGE_CURVE('',#18329,#18330,#17056,.T.);
#22636=EDGE_CURVE('',#18330,#18331,#7861,.T.);
#22637=EDGE_CURVE('',#18331,#18332,#17057,.T.);
#22638=EDGE_CURVE('',#18332,#18333,#7862,.T.);
#22639=EDGE_CURVE('',#18333,#18334,#17058,.T.);
#22640=EDGE_CURVE('',#18334,#18335,#7863,.T.);
#22641=EDGE_CURVE('',#18335,#18328,#17059,.T.);
#22642=EDGE_CURVE('',#18336,#18337,#17060,.T.);
#22643=EDGE_CURVE('',#18338,#18337,#7864,.T.);
#22644=EDGE_CURVE('',#18339,#18338,#17061,.T.);
#22645=EDGE_CURVE('',#18340,#18339,#7865,.T.);
#22646=EDGE_CURVE('',#18340,#18341,#17062,.T.);
#22647=EDGE_CURVE('',#18341,#18342,#7866,.T.);
#22648=EDGE_CURVE('',#18343,#18342,#17063,.T.);
#22649=EDGE_CURVE('',#18344,#18343,#7867,.T.);
#22650=EDGE_CURVE('',#18344,#18345,#17064,.T.);
#22651=EDGE_CURVE('',#18345,#18346,#7868,.T.);
#22652=EDGE_CURVE('',#18347,#18346,#17065,.T.);
#22653=EDGE_CURVE('',#18347,#18336,#7869,.T.);
#22654=EDGE_CURVE('',#18348,#18253,#7870,.T.);
#22655=EDGE_CURVE('',#18348,#18349,#17066,.T.);
#22656=EDGE_CURVE('',#18349,#18350,#7871,.T.);
#22657=EDGE_CURVE('',#18351,#18350,#17067,.T.);
#22658=EDGE_CURVE('',#18351,#18352,#7872,.T.);
#22659=EDGE_CURVE('',#18352,#18353,#17068,.T.);
#22660=EDGE_CURVE('',#18353,#18354,#7873,.T.);
#22661=EDGE_CURVE('',#18354,#18355,#17069,.T.);
#22662=EDGE_CURVE('',#18355,#18356,#7874,.T.);
#22663=EDGE_CURVE('',#18356,#18357,#17070,.T.);
#22664=EDGE_CURVE('',#18254,#18357,#7875,.T.);
#22665=EDGE_CURVE('',#18358,#18359,#7876,.T.);
#22666=EDGE_CURVE('',#18360,#18358,#17071,.T.);
#22667=EDGE_CURVE('',#18360,#18361,#7877,.T.);
#22668=EDGE_CURVE('',#18361,#18362,#17072,.T.);
#22669=EDGE_CURVE('',#18362,#18363,#7878,.T.);
#22670=EDGE_CURVE('',#18364,#18363,#17073,.T.);
#22671=EDGE_CURVE('',#18365,#18364,#7879,.T.);
#22672=EDGE_CURVE('',#18365,#18366,#17074,.T.);
#22673=EDGE_CURVE('',#18367,#18366,#7880,.T.);
#22674=EDGE_CURVE('',#18368,#18367,#17075,.T.);
#22675=EDGE_CURVE('',#18368,#18369,#7881,.T.);
#22676=EDGE_CURVE('',#18369,#18359,#17076,.T.);
#22677=EDGE_CURVE('',#18370,#18371,#7882,.T.);
#22678=EDGE_CURVE('',#18370,#18372,#17077,.T.);
#22679=EDGE_CURVE('',#18372,#18349,#7883,.T.);
#22680=EDGE_CURVE('',#18373,#18348,#7884,.T.);
#22681=EDGE_CURVE('',#18371,#18373,#17078,.T.);
#22682=EDGE_CURVE('',#18374,#18375,#7885,.T.);
#22683=EDGE_CURVE('',#18374,#18370,#7886,.T.);
#22684=EDGE_CURVE('',#18371,#18375,#7887,.T.);
#22685=EDGE_CURVE('',#18376,#18377,#7888,.T.);
#22686=EDGE_CURVE('',#18376,#18378,#17079,.T.);
#22687=EDGE_CURVE('',#18378,#18355,#7889,.T.);
#22688=EDGE_CURVE('',#18379,#18354,#7890,.T.);
#22689=EDGE_CURVE('',#18377,#18379,#17080,.T.);
#22690=EDGE_CURVE('',#18380,#18381,#7891,.T.);
#22691=EDGE_CURVE('',#18380,#18376,#7892,.T.);
#22692=EDGE_CURVE('',#18377,#18381,#7893,.T.);
#22693=EDGE_CURVE('',#18382,#18350,#7894,.T.);
#22694=EDGE_CURVE('',#18382,#18380,#17081,.T.);
#22695=EDGE_CURVE('',#18383,#18381,#17082,.T.);
#22696=EDGE_CURVE('',#18383,#18351,#7895,.T.);
#22697=EDGE_CURVE('',#18372,#18382,#7896,.T.);
#22698=EDGE_CURVE('',#18384,#18356,#7897,.T.);
#22699=EDGE_CURVE('',#18384,#18374,#17083,.T.);
#22700=EDGE_CURVE('',#18385,#18375,#17084,.T.);
#22701=EDGE_CURVE('',#18385,#18357,#7898,.T.);
#22702=EDGE_CURVE('',#18378,#18384,#7899,.T.);
#22703=EDGE_CURVE('',#18386,#18353,#7900,.T.);
#22704=EDGE_CURVE('',#18386,#18379,#7901,.T.);
#22705=EDGE_CURVE('',#18387,#18352,#7902,.T.);
#22706=EDGE_CURVE('',#18387,#18386,#17085,.T.);
#22707=EDGE_CURVE('',#18383,#18387,#7903,.T.);
#22708=EDGE_CURVE('',#18373,#18251,#7904,.T.);
#22709=EDGE_CURVE('',#18252,#18385,#7905,.T.);
#22710=EDGE_CURVE('',#18334,#18382,#17086,.T.);
#22711=EDGE_CURVE('',#18380,#18333,#17087,.T.);
#22712=EDGE_CURVE('',#18376,#18332,#17088,.T.);
#22713=EDGE_CURVE('',#18335,#18372,#17089,.T.);
#22714=EDGE_CURVE('',#18378,#18331,#17090,.T.);
#22715=EDGE_CURVE('',#18328,#18370,#17091,.T.);
#22716=EDGE_CURVE('',#18384,#18330,#17092,.T.);
#22717=EDGE_CURVE('',#18329,#18374,#17093,.T.);
#22718=EDGE_CURVE('',#18257,#18358,#7906,.T.);
#22719=EDGE_CURVE('',#18256,#18360,#7907,.T.);
#22720=EDGE_CURVE('',#18258,#18359,#7908,.T.);
#22721=EDGE_CURVE('',#18259,#18369,#7909,.T.);
#22722=EDGE_CURVE('',#18260,#18368,#7910,.T.);
#22723=EDGE_CURVE('',#18261,#18367,#7911,.T.);
#22724=EDGE_CURVE('',#18262,#18366,#7912,.T.);
#22725=EDGE_CURVE('',#18263,#18365,#7913,.T.);
#22726=EDGE_CURVE('',#18264,#18364,#7914,.T.);
#22727=EDGE_CURVE('',#18265,#18363,#7915,.T.);
#22728=EDGE_CURVE('',#18266,#18362,#7916,.T.);
#22729=EDGE_CURVE('',#18267,#18361,#7917,.T.);
#22730=EDGE_CURVE('',#18316,#18336,#7918,.T.);
#22731=EDGE_CURVE('',#18317,#18337,#7919,.T.);
#22732=EDGE_CURVE('',#18327,#18338,#7920,.T.);
#22733=EDGE_CURVE('',#18326,#18339,#7921,.T.);
#22734=EDGE_CURVE('',#18325,#18340,#7922,.T.);
#22735=EDGE_CURVE('',#18324,#18341,#7923,.T.);
#22736=EDGE_CURVE('',#18323,#18342,#7924,.T.);
#22737=EDGE_CURVE('',#18322,#18343,#7925,.T.);
#22738=EDGE_CURVE('',#18321,#18344,#7926,.T.);
#22739=EDGE_CURVE('',#18320,#18345,#7927,.T.);
#22740=EDGE_CURVE('',#18319,#18346,#7928,.T.);
#22741=EDGE_CURVE('',#18318,#18347,#7929,.T.);
#22742=EDGE_CURVE('',#18289,#18285,#7930,.T.);
#22743=EDGE_CURVE('',#18314,#18311,#7931,.T.);
#22744=EDGE_CURVE('',#18302,#18295,#7932,.T.);
#22745=EDGE_CURVE('',#18388,#18389,#7933,.T.);
#22746=EDGE_CURVE('',#18390,#18389,#7934,.T.);
#22747=EDGE_CURVE('',#18390,#18391,#7935,.T.);
#22748=EDGE_CURVE('',#18388,#18391,#7936,.T.);
#22749=EDGE_CURVE('',#18392,#18393,#7937,.T.);
#22750=EDGE_CURVE('',#18393,#18394,#7938,.T.);
#22751=EDGE_CURVE('',#18394,#18395,#7939,.T.);
#22752=EDGE_CURVE('',#18392,#18395,#7940,.T.);
#22753=EDGE_CURVE('',#18389,#18269,#7941,.T.);
#22754=EDGE_CURVE('',#18388,#18270,#7942,.T.);
#22755=EDGE_CURVE('',#18390,#18268,#7943,.T.);
#22756=EDGE_CURVE('',#18391,#18271,#7944,.T.);
#22757=EDGE_CURVE('',#18396,#18397,#7945,.T.);
#22758=EDGE_CURVE('',#18397,#18398,#7946,.T.);
#22759=EDGE_CURVE('',#18399,#18398,#7947,.T.);
#22760=EDGE_CURVE('',#18399,#18396,#7948,.T.);
#22761=EDGE_CURVE('',#18400,#18399,#7949,.T.);
#22762=EDGE_CURVE('',#18400,#18401,#7950,.T.);
#22763=EDGE_CURVE('',#18401,#18396,#7951,.T.);
#22764=EDGE_CURVE('',#18401,#18402,#7952,.T.);
#22765=EDGE_CURVE('',#18400,#18403,#7953,.T.);
#22766=EDGE_CURVE('',#18402,#18403,#7954,.T.);
#22767=EDGE_CURVE('',#18402,#18394,#7955,.T.);
#22768=EDGE_CURVE('',#18403,#18395,#7956,.T.);
#22769=EDGE_CURVE('',#18398,#18392,#7957,.T.);
#22770=EDGE_CURVE('',#18397,#18393,#7958,.T.);
#22771=EDGE_CURVE('',#18404,#18276,#7959,.T.);
#22772=EDGE_CURVE('',#18404,#18405,#7960,.T.);
#22773=EDGE_CURVE('',#18405,#18277,#7961,.T.);
#22774=EDGE_CURVE('',#18406,#18279,#7962,.T.);
#22775=EDGE_CURVE('',#18404,#18406,#7963,.T.);
#22776=EDGE_CURVE('',#18407,#18278,#7964,.T.);
#22777=EDGE_CURVE('',#18407,#18406,#7965,.T.);
#22778=EDGE_CURVE('',#18407,#18405,#7966,.T.);
#22779=EDGE_CURVE('',#18408,#18409,#7967,.T.);
#22780=EDGE_CURVE('',#18408,#18410,#7968,.T.);
#22781=EDGE_CURVE('',#18410,#18411,#7969,.T.);
#22782=EDGE_CURVE('',#18411,#18409,#7970,.T.);
#22783=EDGE_CURVE('',#18412,#18413,#7971,.T.);
#22784=EDGE_CURVE('',#18413,#18414,#7972,.T.);
#22785=EDGE_CURVE('',#18415,#18414,#7973,.T.);
#22786=EDGE_CURVE('',#18412,#18415,#7974,.T.);
#22787=EDGE_CURVE('',#18412,#18416,#7975,.T.);
#22788=EDGE_CURVE('',#18417,#18415,#7976,.T.);
#22789=EDGE_CURVE('',#18416,#18417,#7977,.T.);
#22790=EDGE_CURVE('',#18418,#18419,#7978,.T.);
#22791=EDGE_CURVE('',#18419,#18414,#7979,.T.);
#22792=EDGE_CURVE('',#18413,#18418,#7980,.T.);
#22793=EDGE_CURVE('',#18419,#18411,#7981,.T.);
#22794=EDGE_CURVE('',#18418,#18409,#7982,.T.);
#22795=EDGE_CURVE('',#18416,#18408,#7983,.T.);
#22796=EDGE_CURVE('',#18417,#18410,#7984,.T.);
#22797=EDGE_CURVE('',#18420,#18421,#7985,.T.);
#22798=EDGE_CURVE('',#18420,#18422,#7986,.T.);
#22799=EDGE_CURVE('',#18423,#18422,#7987,.T.);
#22800=EDGE_CURVE('',#18423,#18421,#7988,.T.);
#22801=EDGE_CURVE('',#18424,#18425,#7989,.T.);
#22802=EDGE_CURVE('',#18424,#18426,#7990,.T.);
#22803=EDGE_CURVE('',#18426,#18427,#7991,.T.);
#22804=EDGE_CURVE('',#18427,#18425,#7992,.T.);
#22805=EDGE_CURVE('',#18420,#18272,#7993,.T.);
#22806=EDGE_CURVE('',#18421,#18273,#7994,.T.);
#22807=EDGE_CURVE('',#18422,#18275,#7995,.T.);
#22808=EDGE_CURVE('',#18423,#18274,#7996,.T.);
#22809=EDGE_CURVE('',#18428,#18429,#7997,.T.);
#22810=EDGE_CURVE('',#18428,#18430,#7998,.T.);
#22811=EDGE_CURVE('',#18430,#18431,#7999,.T.);
#22812=EDGE_CURVE('',#18429,#18431,#8000,.T.);
#22813=EDGE_CURVE('',#18432,#18433,#8001,.T.);
#22814=EDGE_CURVE('',#18431,#18433,#8002,.T.);
#22815=EDGE_CURVE('',#18430,#18432,#8003,.T.);
#22816=EDGE_CURVE('',#18429,#18434,#8004,.T.);
#22817=EDGE_CURVE('',#18435,#18434,#8005,.T.);
#22818=EDGE_CURVE('',#18428,#18435,#8006,.T.);
#22819=EDGE_CURVE('',#18435,#18427,#8007,.T.);
#22820=EDGE_CURVE('',#18434,#18425,#8008,.T.);
#22821=EDGE_CURVE('',#18433,#18424,#8009,.T.);
#22822=EDGE_CURVE('',#18432,#18426,#8010,.T.);
#29809=ORIENTED_EDGE('',*,*,#22522,.F.);
#29810=ORIENTED_EDGE('',*,*,#22523,.T.);
#29811=ORIENTED_EDGE('',*,*,#22524,.T.);
#29812=ORIENTED_EDGE('',*,*,#22523,.F.);
#29813=ORIENTED_EDGE('',*,*,#22525,.T.);
#29814=ORIENTED_EDGE('',*,*,#22526,.T.);
#29815=ORIENTED_EDGE('',*,*,#22527,.T.);
#29816=ORIENTED_EDGE('',*,*,#22526,.F.);
#29817=ORIENTED_EDGE('',*,*,#22528,.T.);
#29818=ORIENTED_EDGE('',*,*,#22529,.T.);
#29819=ORIENTED_EDGE('',*,*,#22530,.F.);
#29820=ORIENTED_EDGE('',*,*,#22529,.F.);
#29821=ORIENTED_EDGE('',*,*,#22531,.F.);
#29822=ORIENTED_EDGE('',*,*,#22532,.F.);
#29823=ORIENTED_EDGE('',*,*,#22533,.T.);
#29824=ORIENTED_EDGE('',*,*,#22534,.F.);
#29825=ORIENTED_EDGE('',*,*,#22533,.F.);
#29826=ORIENTED_EDGE('',*,*,#22535,.F.);
#29827=ORIENTED_EDGE('',*,*,#22536,.F.);
#29828=ORIENTED_EDGE('',*,*,#22537,.T.);
#29829=ORIENTED_EDGE('',*,*,#22538,.F.);
#29830=ORIENTED_EDGE('',*,*,#22537,.F.);
#29831=ORIENTED_EDGE('',*,*,#22531,.T.);
#29832=ORIENTED_EDGE('',*,*,#22532,.T.);
#29833=ORIENTED_EDGE('',*,*,#22539,.T.);
#29834=ORIENTED_EDGE('',*,*,#22540,.T.);
#29835=ORIENTED_EDGE('',*,*,#22539,.F.);
#29836=ORIENTED_EDGE('',*,*,#22541,.F.);
#29837=ORIENTED_EDGE('',*,*,#22542,.T.);
#29838=ORIENTED_EDGE('',*,*,#22543,.T.);
#29839=ORIENTED_EDGE('',*,*,#22544,.F.);
#29840=ORIENTED_EDGE('',*,*,#22535,.T.);
#29841=ORIENTED_EDGE('',*,*,#22536,.T.);
#29842=ORIENTED_EDGE('',*,*,#22545,.T.);
#29843=ORIENTED_EDGE('',*,*,#22546,.T.);
#29844=ORIENTED_EDGE('',*,*,#22545,.F.);
#29845=ORIENTED_EDGE('',*,*,#22547,.T.);
#29846=ORIENTED_EDGE('',*,*,#22548,.T.);
#29847=ORIENTED_EDGE('',*,*,#22549,.F.);
#29848=ORIENTED_EDGE('',*,*,#22550,.F.);
#29849=ORIENTED_EDGE('',*,*,#22551,.T.);
#29850=ORIENTED_EDGE('',*,*,#22552,.T.);
#29851=ORIENTED_EDGE('',*,*,#22553,.F.);
#29852=ORIENTED_EDGE('',*,*,#22554,.T.);
#29853=ORIENTED_EDGE('',*,*,#22555,.T.);
#29854=ORIENTED_EDGE('',*,*,#22556,.F.);
#29855=ORIENTED_EDGE('',*,*,#22557,.F.);
#29856=ORIENTED_EDGE('',*,*,#22558,.F.);
#29857=ORIENTED_EDGE('',*,*,#22559,.T.);
#29858=ORIENTED_EDGE('',*,*,#22560,.F.);
#29859=ORIENTED_EDGE('',*,*,#22561,.T.);
#29860=ORIENTED_EDGE('',*,*,#22562,.F.);
#29861=ORIENTED_EDGE('',*,*,#22563,.T.);
#29862=ORIENTED_EDGE('',*,*,#22564,.F.);
#29863=ORIENTED_EDGE('',*,*,#22565,.T.);
#29864=ORIENTED_EDGE('',*,*,#22566,.F.);
#29865=ORIENTED_EDGE('',*,*,#22567,.T.);
#29866=ORIENTED_EDGE('',*,*,#22568,.F.);
#29867=ORIENTED_EDGE('',*,*,#22569,.T.);
#29868=ORIENTED_EDGE('',*,*,#22570,.F.);
#29869=ORIENTED_EDGE('',*,*,#22571,.F.);
#29870=ORIENTED_EDGE('',*,*,#22572,.T.);
#29871=ORIENTED_EDGE('',*,*,#22573,.T.);
#29872=ORIENTED_EDGE('',*,*,#22574,.F.);
#29873=ORIENTED_EDGE('',*,*,#22575,.F.);
#29874=ORIENTED_EDGE('',*,*,#22576,.T.);
#29875=ORIENTED_EDGE('',*,*,#22577,.T.);
#29876=ORIENTED_EDGE('',*,*,#22574,.T.);
#29877=ORIENTED_EDGE('',*,*,#22578,.F.);
#29878=ORIENTED_EDGE('',*,*,#22579,.F.);
#29879=ORIENTED_EDGE('',*,*,#22580,.T.);
#29880=ORIENTED_EDGE('',*,*,#22581,.T.);
#29881=ORIENTED_EDGE('',*,*,#22582,.F.);
#29882=ORIENTED_EDGE('',*,*,#22572,.F.);
#29883=ORIENTED_EDGE('',*,*,#22583,.F.);
#29884=ORIENTED_EDGE('',*,*,#22584,.T.);
#29885=ORIENTED_EDGE('',*,*,#22576,.F.);
#29886=ORIENTED_EDGE('',*,*,#22585,.T.);
#29887=ORIENTED_EDGE('',*,*,#22584,.F.);
#29888=ORIENTED_EDGE('',*,*,#22586,.F.);
#29889=ORIENTED_EDGE('',*,*,#22587,.F.);
#29890=ORIENTED_EDGE('',*,*,#22588,.F.);
#29891=ORIENTED_EDGE('',*,*,#22589,.T.);
#29892=ORIENTED_EDGE('',*,*,#22590,.T.);
#29893=ORIENTED_EDGE('',*,*,#22591,.T.);
#29894=ORIENTED_EDGE('',*,*,#22592,.F.);
#29895=ORIENTED_EDGE('',*,*,#22593,.F.);
#29896=ORIENTED_EDGE('',*,*,#22594,.T.);
#29897=ORIENTED_EDGE('',*,*,#22592,.T.);
#29898=ORIENTED_EDGE('',*,*,#22595,.F.);
#29899=ORIENTED_EDGE('',*,*,#22596,.T.);
#29900=ORIENTED_EDGE('',*,*,#22593,.T.);
#29901=ORIENTED_EDGE('',*,*,#22597,.T.);
#29902=ORIENTED_EDGE('',*,*,#22598,.F.);
#29903=ORIENTED_EDGE('',*,*,#22599,.F.);
#29904=ORIENTED_EDGE('',*,*,#22600,.F.);
#29905=ORIENTED_EDGE('',*,*,#22588,.T.);
#29906=ORIENTED_EDGE('',*,*,#22601,.T.);
#29907=ORIENTED_EDGE('',*,*,#22600,.T.);
#29908=ORIENTED_EDGE('',*,*,#22602,.F.);
#29909=ORIENTED_EDGE('',*,*,#22603,.F.);
#29910=ORIENTED_EDGE('',*,*,#22604,.T.);
#29911=ORIENTED_EDGE('',*,*,#22605,.T.);
#29912=ORIENTED_EDGE('',*,*,#22606,.F.);
#29913=ORIENTED_EDGE('',*,*,#22607,.T.);
#29914=ORIENTED_EDGE('',*,*,#22608,.T.);
#29915=ORIENTED_EDGE('',*,*,#22606,.T.);
#29916=ORIENTED_EDGE('',*,*,#22609,.F.);
#29917=ORIENTED_EDGE('',*,*,#22610,.F.);
#29918=ORIENTED_EDGE('',*,*,#22611,.F.);
#29919=ORIENTED_EDGE('',*,*,#22604,.F.);
#29920=ORIENTED_EDGE('',*,*,#22612,.T.);
#29921=ORIENTED_EDGE('',*,*,#22613,.T.);
#29922=ORIENTED_EDGE('',*,*,#22614,.F.);
#29923=ORIENTED_EDGE('',*,*,#22615,.T.);
#29924=ORIENTED_EDGE('',*,*,#22616,.F.);
#29925=ORIENTED_EDGE('',*,*,#22617,.F.);
#29926=ORIENTED_EDGE('',*,*,#22607,.F.);
#29927=ORIENTED_EDGE('',*,*,#22618,.T.);
#29928=ORIENTED_EDGE('',*,*,#22613,.F.);
#29929=ORIENTED_EDGE('',*,*,#22619,.F.);
#29930=ORIENTED_EDGE('',*,*,#22620,.F.);
#29931=ORIENTED_EDGE('',*,*,#22621,.T.);
#29932=ORIENTED_EDGE('',*,*,#22622,.F.);
#29933=ORIENTED_EDGE('',*,*,#22623,.F.);
#29934=ORIENTED_EDGE('',*,*,#22624,.T.);
#29935=ORIENTED_EDGE('',*,*,#22625,.T.);
#29936=ORIENTED_EDGE('',*,*,#22626,.F.);
#29937=ORIENTED_EDGE('',*,*,#22627,.F.);
#29938=ORIENTED_EDGE('',*,*,#22628,.T.);
#29939=ORIENTED_EDGE('',*,*,#22629,.T.);
#29940=ORIENTED_EDGE('',*,*,#22630,.T.);
#29941=ORIENTED_EDGE('',*,*,#22605,.F.);
#29942=ORIENTED_EDGE('',*,*,#22616,.T.);
#29943=ORIENTED_EDGE('',*,*,#22631,.F.);
#29944=ORIENTED_EDGE('',*,*,#22609,.T.);
#29945=ORIENTED_EDGE('',*,*,#22591,.F.);
#29946=ORIENTED_EDGE('',*,*,#22632,.T.);
#29947=ORIENTED_EDGE('',*,*,#22597,.F.);
#29948=ORIENTED_EDGE('',*,*,#22595,.T.);
#29949=ORIENTED_EDGE('',*,*,#22573,.F.);
#29950=ORIENTED_EDGE('',*,*,#22582,.T.);
#29951=ORIENTED_EDGE('',*,*,#22633,.F.);
#29952=ORIENTED_EDGE('',*,*,#22578,.T.);
#29953=ORIENTED_EDGE('',*,*,#22634,.T.);
#29954=ORIENTED_EDGE('',*,*,#22635,.T.);
#29955=ORIENTED_EDGE('',*,*,#22636,.T.);
#29956=ORIENTED_EDGE('',*,*,#22637,.T.);
#29957=ORIENTED_EDGE('',*,*,#22638,.T.);
#29958=ORIENTED_EDGE('',*,*,#22639,.T.);
#29959=ORIENTED_EDGE('',*,*,#22640,.T.);
#29960=ORIENTED_EDGE('',*,*,#22641,.T.);
#29961=ORIENTED_EDGE('',*,*,#22642,.T.);
#29962=ORIENTED_EDGE('',*,*,#22643,.F.);
#29963=ORIENTED_EDGE('',*,*,#22644,.F.);
#29964=ORIENTED_EDGE('',*,*,#22645,.F.);
#29965=ORIENTED_EDGE('',*,*,#22646,.T.);
#29966=ORIENTED_EDGE('',*,*,#22647,.T.);
#29967=ORIENTED_EDGE('',*,*,#22648,.F.);
#29968=ORIENTED_EDGE('',*,*,#22649,.F.);
#29969=ORIENTED_EDGE('',*,*,#22650,.T.);
#29970=ORIENTED_EDGE('',*,*,#22651,.T.);
#29971=ORIENTED_EDGE('',*,*,#22652,.F.);
#29972=ORIENTED_EDGE('',*,*,#22653,.T.);
#29973=ORIENTED_EDGE('',*,*,#22654,.F.);
#29974=ORIENTED_EDGE('',*,*,#22655,.T.);
#29975=ORIENTED_EDGE('',*,*,#22656,.T.);
#29976=ORIENTED_EDGE('',*,*,#22657,.F.);
#29977=ORIENTED_EDGE('',*,*,#22658,.T.);
#29978=ORIENTED_EDGE('',*,*,#22659,.T.);
#29979=ORIENTED_EDGE('',*,*,#22660,.T.);
#29980=ORIENTED_EDGE('',*,*,#22661,.T.);
#29981=ORIENTED_EDGE('',*,*,#22662,.T.);
#29982=ORIENTED_EDGE('',*,*,#22663,.T.);
#29983=ORIENTED_EDGE('',*,*,#22664,.F.);
#29984=ORIENTED_EDGE('',*,*,#22543,.F.);
#29985=ORIENTED_EDGE('',*,*,#22546,.F.);
#29986=ORIENTED_EDGE('',*,*,#22540,.F.);
#29987=ORIENTED_EDGE('',*,*,#22665,.F.);
#29988=ORIENTED_EDGE('',*,*,#22666,.F.);
#29989=ORIENTED_EDGE('',*,*,#22667,.T.);
#29990=ORIENTED_EDGE('',*,*,#22668,.T.);
#29991=ORIENTED_EDGE('',*,*,#22669,.T.);
#29992=ORIENTED_EDGE('',*,*,#22670,.F.);
#29993=ORIENTED_EDGE('',*,*,#22671,.F.);
#29994=ORIENTED_EDGE('',*,*,#22672,.T.);
#29995=ORIENTED_EDGE('',*,*,#22673,.F.);
#29996=ORIENTED_EDGE('',*,*,#22674,.F.);
#29997=ORIENTED_EDGE('',*,*,#22675,.T.);
#29998=ORIENTED_EDGE('',*,*,#22676,.T.);
#29999=ORIENTED_EDGE('',*,*,#22677,.F.);
#30000=ORIENTED_EDGE('',*,*,#22678,.T.);
#30001=ORIENTED_EDGE('',*,*,#22679,.T.);
#30002=ORIENTED_EDGE('',*,*,#22655,.F.);
#30003=ORIENTED_EDGE('',*,*,#22680,.F.);
#30004=ORIENTED_EDGE('',*,*,#22681,.F.);
#30005=ORIENTED_EDGE('',*,*,#22682,.F.);
#30006=ORIENTED_EDGE('',*,*,#22683,.T.);
#30007=ORIENTED_EDGE('',*,*,#22677,.T.);
#30008=ORIENTED_EDGE('',*,*,#22684,.T.);
#30009=ORIENTED_EDGE('',*,*,#22685,.F.);
#30010=ORIENTED_EDGE('',*,*,#22686,.T.);
#30011=ORIENTED_EDGE('',*,*,#22687,.T.);
#30012=ORIENTED_EDGE('',*,*,#22661,.F.);
#30013=ORIENTED_EDGE('',*,*,#22688,.F.);
#30014=ORIENTED_EDGE('',*,*,#22689,.F.);
#30015=ORIENTED_EDGE('',*,*,#22690,.F.);
#30016=ORIENTED_EDGE('',*,*,#22691,.T.);
#30017=ORIENTED_EDGE('',*,*,#22685,.T.);
#30018=ORIENTED_EDGE('',*,*,#22692,.T.);
#30019=ORIENTED_EDGE('',*,*,#22693,.F.);
#30020=ORIENTED_EDGE('',*,*,#22694,.T.);
#30021=ORIENTED_EDGE('',*,*,#22690,.T.);
#30022=ORIENTED_EDGE('',*,*,#22695,.F.);
#30023=ORIENTED_EDGE('',*,*,#22696,.T.);
#30024=ORIENTED_EDGE('',*,*,#22657,.T.);
#30025=ORIENTED_EDGE('',*,*,#22679,.F.);
#30026=ORIENTED_EDGE('',*,*,#22697,.T.);
#30027=ORIENTED_EDGE('',*,*,#22693,.T.);
#30028=ORIENTED_EDGE('',*,*,#22656,.F.);
#30029=ORIENTED_EDGE('',*,*,#22698,.F.);
#30030=ORIENTED_EDGE('',*,*,#22699,.T.);
#30031=ORIENTED_EDGE('',*,*,#22682,.T.);
#30032=ORIENTED_EDGE('',*,*,#22700,.F.);
#30033=ORIENTED_EDGE('',*,*,#22701,.T.);
#30034=ORIENTED_EDGE('',*,*,#22663,.F.);
#30035=ORIENTED_EDGE('',*,*,#22687,.F.);
#30036=ORIENTED_EDGE('',*,*,#22702,.T.);
#30037=ORIENTED_EDGE('',*,*,#22698,.T.);
#30038=ORIENTED_EDGE('',*,*,#22662,.F.);
#30039=ORIENTED_EDGE('',*,*,#22660,.F.);
#30040=ORIENTED_EDGE('',*,*,#22703,.F.);
#30041=ORIENTED_EDGE('',*,*,#22704,.T.);
#30042=ORIENTED_EDGE('',*,*,#22688,.T.);
#30043=ORIENTED_EDGE('',*,*,#22659,.F.);
#30044=ORIENTED_EDGE('',*,*,#22705,.F.);
#30045=ORIENTED_EDGE('',*,*,#22706,.T.);
#30046=ORIENTED_EDGE('',*,*,#22703,.T.);
#30047=ORIENTED_EDGE('',*,*,#22658,.F.);
#30048=ORIENTED_EDGE('',*,*,#22696,.F.);
#30049=ORIENTED_EDGE('',*,*,#22707,.T.);
#30050=ORIENTED_EDGE('',*,*,#22705,.T.);
#30051=ORIENTED_EDGE('',*,*,#22695,.T.);
#30052=ORIENTED_EDGE('',*,*,#22692,.F.);
#30053=ORIENTED_EDGE('',*,*,#22689,.T.);
#30054=ORIENTED_EDGE('',*,*,#22704,.F.);
#30055=ORIENTED_EDGE('',*,*,#22706,.F.);
#30056=ORIENTED_EDGE('',*,*,#22707,.F.);
#30057=ORIENTED_EDGE('',*,*,#22538,.T.);
#30058=ORIENTED_EDGE('',*,*,#22654,.T.);
#30059=ORIENTED_EDGE('',*,*,#22542,.F.);
#30060=ORIENTED_EDGE('',*,*,#22708,.F.);
#30061=ORIENTED_EDGE('',*,*,#22680,.T.);
#30062=ORIENTED_EDGE('',*,*,#22664,.T.);
#30063=ORIENTED_EDGE('',*,*,#22701,.F.);
#30064=ORIENTED_EDGE('',*,*,#22709,.F.);
#30065=ORIENTED_EDGE('',*,*,#22544,.T.);
#30066=ORIENTED_EDGE('',*,*,#22681,.T.);
#30067=ORIENTED_EDGE('',*,*,#22708,.T.);
#30068=ORIENTED_EDGE('',*,*,#22541,.T.);
#30069=ORIENTED_EDGE('',*,*,#22709,.T.);
#30070=ORIENTED_EDGE('',*,*,#22700,.T.);
#30071=ORIENTED_EDGE('',*,*,#22684,.F.);
#30072=ORIENTED_EDGE('',*,*,#22534,.T.);
#30073=ORIENTED_EDGE('',*,*,#22710,.F.);
#30074=ORIENTED_EDGE('',*,*,#22639,.F.);
#30075=ORIENTED_EDGE('',*,*,#22711,.F.);
#30076=ORIENTED_EDGE('',*,*,#22694,.F.);
#30077=ORIENTED_EDGE('',*,*,#22711,.T.);
#30078=ORIENTED_EDGE('',*,*,#22638,.F.);
#30079=ORIENTED_EDGE('',*,*,#22712,.F.);
#30080=ORIENTED_EDGE('',*,*,#22691,.F.);
#30081=ORIENTED_EDGE('',*,*,#22710,.T.);
#30082=ORIENTED_EDGE('',*,*,#22697,.F.);
#30083=ORIENTED_EDGE('',*,*,#22713,.F.);
#30084=ORIENTED_EDGE('',*,*,#22640,.F.);
#30085=ORIENTED_EDGE('',*,*,#22712,.T.);
#30086=ORIENTED_EDGE('',*,*,#22637,.F.);
#30087=ORIENTED_EDGE('',*,*,#22714,.F.);
#30088=ORIENTED_EDGE('',*,*,#22686,.F.);
#30089=ORIENTED_EDGE('',*,*,#22713,.T.);
#30090=ORIENTED_EDGE('',*,*,#22678,.F.);
#30091=ORIENTED_EDGE('',*,*,#22715,.F.);
#30092=ORIENTED_EDGE('',*,*,#22641,.F.);
#30093=ORIENTED_EDGE('',*,*,#22714,.T.);
#30094=ORIENTED_EDGE('',*,*,#22636,.F.);
#30095=ORIENTED_EDGE('',*,*,#22716,.F.);
#30096=ORIENTED_EDGE('',*,*,#22702,.F.);
#30097=ORIENTED_EDGE('',*,*,#22715,.T.);
#30098=ORIENTED_EDGE('',*,*,#22683,.F.);
#30099=ORIENTED_EDGE('',*,*,#22717,.F.);
#30100=ORIENTED_EDGE('',*,*,#22634,.F.);
#30101=ORIENTED_EDGE('',*,*,#22716,.T.);
#30102=ORIENTED_EDGE('',*,*,#22635,.F.);
#30103=ORIENTED_EDGE('',*,*,#22717,.T.);
#30104=ORIENTED_EDGE('',*,*,#22699,.F.);
#30105=ORIENTED_EDGE('',*,*,#22666,.T.);
#30106=ORIENTED_EDGE('',*,*,#22718,.F.);
#30107=ORIENTED_EDGE('',*,*,#22547,.F.);
#30108=ORIENTED_EDGE('',*,*,#22719,.T.);
#30109=ORIENTED_EDGE('',*,*,#22665,.T.);
#30110=ORIENTED_EDGE('',*,*,#22720,.F.);
#30111=ORIENTED_EDGE('',*,*,#22548,.F.);
#30112=ORIENTED_EDGE('',*,*,#22718,.T.);
#30113=ORIENTED_EDGE('',*,*,#22676,.F.);
#30114=ORIENTED_EDGE('',*,*,#22721,.F.);
#30115=ORIENTED_EDGE('',*,*,#22549,.T.);
#30116=ORIENTED_EDGE('',*,*,#22720,.T.);
#30117=ORIENTED_EDGE('',*,*,#22675,.F.);
#30118=ORIENTED_EDGE('',*,*,#22722,.F.);
#30119=ORIENTED_EDGE('',*,*,#22550,.T.);
#30120=ORIENTED_EDGE('',*,*,#22721,.T.);
#30121=ORIENTED_EDGE('',*,*,#22674,.T.);
#30122=ORIENTED_EDGE('',*,*,#22723,.F.);
#30123=ORIENTED_EDGE('',*,*,#22551,.F.);
#30124=ORIENTED_EDGE('',*,*,#22722,.T.);
#30125=ORIENTED_EDGE('',*,*,#22673,.T.);
#30126=ORIENTED_EDGE('',*,*,#22724,.F.);
#30127=ORIENTED_EDGE('',*,*,#22552,.F.);
#30128=ORIENTED_EDGE('',*,*,#22723,.T.);
#30129=ORIENTED_EDGE('',*,*,#22672,.F.);
#30130=ORIENTED_EDGE('',*,*,#22725,.F.);
#30131=ORIENTED_EDGE('',*,*,#22553,.T.);
#30132=ORIENTED_EDGE('',*,*,#22724,.T.);
#30133=ORIENTED_EDGE('',*,*,#22671,.T.);
#30134=ORIENTED_EDGE('',*,*,#22726,.F.);
#30135=ORIENTED_EDGE('',*,*,#22554,.F.);
#30136=ORIENTED_EDGE('',*,*,#22725,.T.);
#30137=ORIENTED_EDGE('',*,*,#22670,.T.);
#30138=ORIENTED_EDGE('',*,*,#22727,.F.);
#30139=ORIENTED_EDGE('',*,*,#22555,.F.);
#30140=ORIENTED_EDGE('',*,*,#22726,.T.);
#30141=ORIENTED_EDGE('',*,*,#22669,.F.);
#30142=ORIENTED_EDGE('',*,*,#22728,.F.);
#30143=ORIENTED_EDGE('',*,*,#22556,.T.);
#30144=ORIENTED_EDGE('',*,*,#22727,.T.);
#30145=ORIENTED_EDGE('',*,*,#22668,.F.);
#30146=ORIENTED_EDGE('',*,*,#22729,.F.);
#30147=ORIENTED_EDGE('',*,*,#22557,.T.);
#30148=ORIENTED_EDGE('',*,*,#22728,.T.);
#30149=ORIENTED_EDGE('',*,*,#22667,.F.);
#30150=ORIENTED_EDGE('',*,*,#22719,.F.);
#30151=ORIENTED_EDGE('',*,*,#22558,.T.);
#30152=ORIENTED_EDGE('',*,*,#22729,.T.);
#30153=ORIENTED_EDGE('',*,*,#22642,.F.);
#30154=ORIENTED_EDGE('',*,*,#22730,.F.);
#30155=ORIENTED_EDGE('',*,*,#22619,.T.);
#30156=ORIENTED_EDGE('',*,*,#22731,.T.);
#30157=ORIENTED_EDGE('',*,*,#22643,.T.);
#30158=ORIENTED_EDGE('',*,*,#22731,.F.);
#30159=ORIENTED_EDGE('',*,*,#22630,.F.);
#30160=ORIENTED_EDGE('',*,*,#22732,.T.);
#30161=ORIENTED_EDGE('',*,*,#22644,.T.);
#30162=ORIENTED_EDGE('',*,*,#22732,.F.);
#30163=ORIENTED_EDGE('',*,*,#22629,.F.);
#30164=ORIENTED_EDGE('',*,*,#22733,.T.);
#30165=ORIENTED_EDGE('',*,*,#22645,.T.);
#30166=ORIENTED_EDGE('',*,*,#22733,.F.);
#30167=ORIENTED_EDGE('',*,*,#22628,.F.);
#30168=ORIENTED_EDGE('',*,*,#22734,.T.);
#30169=ORIENTED_EDGE('',*,*,#22646,.F.);
#30170=ORIENTED_EDGE('',*,*,#22734,.F.);
#30171=ORIENTED_EDGE('',*,*,#22627,.T.);
#30172=ORIENTED_EDGE('',*,*,#22735,.T.);
#30173=ORIENTED_EDGE('',*,*,#22647,.F.);
#30174=ORIENTED_EDGE('',*,*,#22735,.F.);
#30175=ORIENTED_EDGE('',*,*,#22626,.T.);
#30176=ORIENTED_EDGE('',*,*,#22736,.T.);
#30177=ORIENTED_EDGE('',*,*,#22648,.T.);
#30178=ORIENTED_EDGE('',*,*,#22736,.F.);
#30179=ORIENTED_EDGE('',*,*,#22625,.F.);
#30180=ORIENTED_EDGE('',*,*,#22737,.T.);
#30181=ORIENTED_EDGE('',*,*,#22649,.T.);
#30182=ORIENTED_EDGE('',*,*,#22737,.F.);
#30183=ORIENTED_EDGE('',*,*,#22624,.F.);
#30184=ORIENTED_EDGE('',*,*,#22738,.T.);
#30185=ORIENTED_EDGE('',*,*,#22650,.F.);
#30186=ORIENTED_EDGE('',*,*,#22738,.F.);
#30187=ORIENTED_EDGE('',*,*,#22623,.T.);
#30188=ORIENTED_EDGE('',*,*,#22739,.T.);
#30189=ORIENTED_EDGE('',*,*,#22651,.F.);
#30190=ORIENTED_EDGE('',*,*,#22739,.F.);
#30191=ORIENTED_EDGE('',*,*,#22622,.T.);
#30192=ORIENTED_EDGE('',*,*,#22740,.T.);
#30193=ORIENTED_EDGE('',*,*,#22652,.T.);
#30194=ORIENTED_EDGE('',*,*,#22740,.F.);
#30195=ORIENTED_EDGE('',*,*,#22621,.F.);
#30196=ORIENTED_EDGE('',*,*,#22741,.T.);
#30197=ORIENTED_EDGE('',*,*,#22653,.F.);
#30198=ORIENTED_EDGE('',*,*,#22741,.F.);
#30199=ORIENTED_EDGE('',*,*,#22620,.T.);
#30200=ORIENTED_EDGE('',*,*,#22730,.T.);
#30201=ORIENTED_EDGE('',*,*,#22581,.F.);
#30202=ORIENTED_EDGE('',*,*,#22742,.T.);
#30203=ORIENTED_EDGE('',*,*,#22579,.T.);
#30204=ORIENTED_EDGE('',*,*,#22633,.T.);
#30205=ORIENTED_EDGE('',*,*,#22615,.F.);
#30206=ORIENTED_EDGE('',*,*,#22743,.T.);
#30207=ORIENTED_EDGE('',*,*,#22610,.T.);
#30208=ORIENTED_EDGE('',*,*,#22631,.T.);
#30209=ORIENTED_EDGE('',*,*,#22744,.F.);
#30210=ORIENTED_EDGE('',*,*,#22598,.T.);
#30211=ORIENTED_EDGE('',*,*,#22632,.F.);
#30212=ORIENTED_EDGE('',*,*,#22590,.F.);
#30213=ORIENTED_EDGE('',*,*,#22614,.T.);
#30214=ORIENTED_EDGE('',*,*,#22618,.F.);
#30215=ORIENTED_EDGE('',*,*,#22611,.T.);
#30216=ORIENTED_EDGE('',*,*,#22743,.F.);
#30217=ORIENTED_EDGE('',*,*,#22603,.T.);
#30218=ORIENTED_EDGE('',*,*,#22608,.F.);
#30219=ORIENTED_EDGE('',*,*,#22617,.T.);
#30220=ORIENTED_EDGE('',*,*,#22612,.F.);
#30221=ORIENTED_EDGE('',*,*,#22744,.T.);
#30222=ORIENTED_EDGE('',*,*,#22589,.F.);
#30223=ORIENTED_EDGE('',*,*,#22602,.T.);
#30224=ORIENTED_EDGE('',*,*,#22599,.T.);
#30225=ORIENTED_EDGE('',*,*,#22596,.F.);
#30226=ORIENTED_EDGE('',*,*,#22601,.F.);
#30227=ORIENTED_EDGE('',*,*,#22587,.T.);
#30228=ORIENTED_EDGE('',*,*,#22594,.F.);
#30229=ORIENTED_EDGE('',*,*,#22571,.T.);
#30230=ORIENTED_EDGE('',*,*,#22577,.F.);
#30231=ORIENTED_EDGE('',*,*,#22586,.T.);
#30232=ORIENTED_EDGE('',*,*,#22583,.T.);
#30233=ORIENTED_EDGE('',*,*,#22580,.F.);
#30234=ORIENTED_EDGE('',*,*,#22585,.F.);
#30235=ORIENTED_EDGE('',*,*,#22575,.T.);
#30236=ORIENTED_EDGE('',*,*,#22742,.F.);
#30237=ORIENTED_EDGE('',*,*,#22745,.T.);
#30238=ORIENTED_EDGE('',*,*,#22746,.F.);
#30239=ORIENTED_EDGE('',*,*,#22747,.T.);
#30240=ORIENTED_EDGE('',*,*,#22748,.F.);
#30241=ORIENTED_EDGE('',*,*,#22749,.T.);
#30242=ORIENTED_EDGE('',*,*,#22750,.T.);
#30243=ORIENTED_EDGE('',*,*,#22751,.T.);
#30244=ORIENTED_EDGE('',*,*,#22752,.F.);
#30245=ORIENTED_EDGE('',*,*,#22560,.T.);
#30246=ORIENTED_EDGE('',*,*,#22753,.F.);
#30247=ORIENTED_EDGE('',*,*,#22745,.F.);
#30248=ORIENTED_EDGE('',*,*,#22754,.T.);
#30249=ORIENTED_EDGE('',*,*,#22559,.F.);
#30250=ORIENTED_EDGE('',*,*,#22755,.F.);
#30251=ORIENTED_EDGE('',*,*,#22746,.T.);
#30252=ORIENTED_EDGE('',*,*,#22753,.T.);
#30253=ORIENTED_EDGE('',*,*,#22562,.T.);
#30254=ORIENTED_EDGE('',*,*,#22756,.F.);
#30255=ORIENTED_EDGE('',*,*,#22747,.F.);
#30256=ORIENTED_EDGE('',*,*,#22755,.T.);
#30257=ORIENTED_EDGE('',*,*,#22561,.F.);
#30258=ORIENTED_EDGE('',*,*,#22754,.F.);
#30259=ORIENTED_EDGE('',*,*,#22748,.T.);
#30260=ORIENTED_EDGE('',*,*,#22756,.T.);
#30261=ORIENTED_EDGE('',*,*,#22757,.T.);
#30262=ORIENTED_EDGE('',*,*,#22758,.T.);
#30263=ORIENTED_EDGE('',*,*,#22759,.F.);
#30264=ORIENTED_EDGE('',*,*,#22760,.T.);
#30265=ORIENTED_EDGE('',*,*,#22761,.F.);
#30266=ORIENTED_EDGE('',*,*,#22762,.T.);
#30267=ORIENTED_EDGE('',*,*,#22763,.T.);
#30268=ORIENTED_EDGE('',*,*,#22760,.F.);
#30269=ORIENTED_EDGE('',*,*,#22764,.F.);
#30270=ORIENTED_EDGE('',*,*,#22762,.F.);
#30271=ORIENTED_EDGE('',*,*,#22765,.T.);
#30272=ORIENTED_EDGE('',*,*,#22766,.F.);
#30273=ORIENTED_EDGE('',*,*,#22751,.F.);
#30274=ORIENTED_EDGE('',*,*,#22767,.F.);
#30275=ORIENTED_EDGE('',*,*,#22766,.T.);
#30276=ORIENTED_EDGE('',*,*,#22768,.T.);
#30277=ORIENTED_EDGE('',*,*,#22769,.T.);
#30278=ORIENTED_EDGE('',*,*,#22752,.T.);
#30279=ORIENTED_EDGE('',*,*,#22768,.F.);
#30280=ORIENTED_EDGE('',*,*,#22765,.F.);
#30281=ORIENTED_EDGE('',*,*,#22761,.T.);
#30282=ORIENTED_EDGE('',*,*,#22759,.T.);
#30283=ORIENTED_EDGE('',*,*,#22530,.T.);
#30284=ORIENTED_EDGE('',*,*,#22749,.F.);
#30285=ORIENTED_EDGE('',*,*,#22769,.F.);
#30286=ORIENTED_EDGE('',*,*,#22758,.F.);
#30287=ORIENTED_EDGE('',*,*,#22770,.T.);
#30288=ORIENTED_EDGE('',*,*,#22750,.F.);
#30289=ORIENTED_EDGE('',*,*,#22770,.F.);
#30290=ORIENTED_EDGE('',*,*,#22757,.F.);
#30291=ORIENTED_EDGE('',*,*,#22763,.F.);
#30292=ORIENTED_EDGE('',*,*,#22764,.T.);
#30293=ORIENTED_EDGE('',*,*,#22767,.T.);
#30294=ORIENTED_EDGE('',*,*,#22528,.F.);
#30295=ORIENTED_EDGE('',*,*,#22567,.F.);
#30296=ORIENTED_EDGE('',*,*,#22771,.F.);
#30297=ORIENTED_EDGE('',*,*,#22772,.T.);
#30298=ORIENTED_EDGE('',*,*,#22773,.T.);
#30299=ORIENTED_EDGE('',*,*,#22570,.T.);
#30300=ORIENTED_EDGE('',*,*,#22774,.F.);
#30301=ORIENTED_EDGE('',*,*,#22775,.F.);
#30302=ORIENTED_EDGE('',*,*,#22771,.T.);
#30303=ORIENTED_EDGE('',*,*,#22569,.F.);
#30304=ORIENTED_EDGE('',*,*,#22776,.F.);
#30305=ORIENTED_EDGE('',*,*,#22777,.T.);
#30306=ORIENTED_EDGE('',*,*,#22774,.T.);
#30307=ORIENTED_EDGE('',*,*,#22568,.T.);
#30308=ORIENTED_EDGE('',*,*,#22773,.F.);
#30309=ORIENTED_EDGE('',*,*,#22778,.F.);
#30310=ORIENTED_EDGE('',*,*,#22776,.T.);
#30311=ORIENTED_EDGE('',*,*,#22772,.F.);
#30312=ORIENTED_EDGE('',*,*,#22775,.T.);
#30313=ORIENTED_EDGE('',*,*,#22777,.F.);
#30314=ORIENTED_EDGE('',*,*,#22778,.T.);
#30315=ORIENTED_EDGE('',*,*,#22779,.F.);
#30316=ORIENTED_EDGE('',*,*,#22780,.T.);
#30317=ORIENTED_EDGE('',*,*,#22781,.T.);
#30318=ORIENTED_EDGE('',*,*,#22782,.T.);
#30319=ORIENTED_EDGE('',*,*,#22783,.T.);
#30320=ORIENTED_EDGE('',*,*,#22784,.T.);
#30321=ORIENTED_EDGE('',*,*,#22785,.F.);
#30322=ORIENTED_EDGE('',*,*,#22786,.F.);
#30323=ORIENTED_EDGE('',*,*,#22787,.F.);
#30324=ORIENTED_EDGE('',*,*,#22786,.T.);
#30325=ORIENTED_EDGE('',*,*,#22788,.F.);
#30326=ORIENTED_EDGE('',*,*,#22789,.F.);
#30327=ORIENTED_EDGE('',*,*,#22790,.T.);
#30328=ORIENTED_EDGE('',*,*,#22791,.T.);
#30329=ORIENTED_EDGE('',*,*,#22784,.F.);
#30330=ORIENTED_EDGE('',*,*,#22792,.T.);
#30331=ORIENTED_EDGE('',*,*,#22782,.F.);
#30332=ORIENTED_EDGE('',*,*,#22793,.F.);
#30333=ORIENTED_EDGE('',*,*,#22790,.F.);
#30334=ORIENTED_EDGE('',*,*,#22794,.T.);
#30335=ORIENTED_EDGE('',*,*,#22780,.F.);
#30336=ORIENTED_EDGE('',*,*,#22795,.F.);
#30337=ORIENTED_EDGE('',*,*,#22789,.T.);
#30338=ORIENTED_EDGE('',*,*,#22796,.T.);
#30339=ORIENTED_EDGE('',*,*,#22781,.F.);
#30340=ORIENTED_EDGE('',*,*,#22796,.F.);
#30341=ORIENTED_EDGE('',*,*,#22788,.T.);
#30342=ORIENTED_EDGE('',*,*,#22785,.T.);
#30343=ORIENTED_EDGE('',*,*,#22791,.F.);
#30344=ORIENTED_EDGE('',*,*,#22793,.T.);
#30345=ORIENTED_EDGE('',*,*,#22525,.F.);
#30346=ORIENTED_EDGE('',*,*,#22795,.T.);
#30347=ORIENTED_EDGE('',*,*,#22779,.T.);
#30348=ORIENTED_EDGE('',*,*,#22794,.F.);
#30349=ORIENTED_EDGE('',*,*,#22792,.F.);
#30350=ORIENTED_EDGE('',*,*,#22783,.F.);
#30351=ORIENTED_EDGE('',*,*,#22787,.T.);
#30352=ORIENTED_EDGE('',*,*,#22527,.F.);
#30353=ORIENTED_EDGE('',*,*,#22797,.F.);
#30354=ORIENTED_EDGE('',*,*,#22798,.T.);
#30355=ORIENTED_EDGE('',*,*,#22799,.F.);
#30356=ORIENTED_EDGE('',*,*,#22800,.T.);
#30357=ORIENTED_EDGE('',*,*,#22801,.F.);
#30358=ORIENTED_EDGE('',*,*,#22802,.T.);
#30359=ORIENTED_EDGE('',*,*,#22803,.T.);
#30360=ORIENTED_EDGE('',*,*,#22804,.T.);
#30361=ORIENTED_EDGE('',*,*,#22563,.F.);
#30362=ORIENTED_EDGE('',*,*,#22805,.F.);
#30363=ORIENTED_EDGE('',*,*,#22797,.T.);
#30364=ORIENTED_EDGE('',*,*,#22806,.T.);
#30365=ORIENTED_EDGE('',*,*,#22566,.T.);
#30366=ORIENTED_EDGE('',*,*,#22807,.F.);
#30367=ORIENTED_EDGE('',*,*,#22798,.F.);
#30368=ORIENTED_EDGE('',*,*,#22805,.T.);
#30369=ORIENTED_EDGE('',*,*,#22565,.F.);
#30370=ORIENTED_EDGE('',*,*,#22808,.F.);
#30371=ORIENTED_EDGE('',*,*,#22799,.T.);
#30372=ORIENTED_EDGE('',*,*,#22807,.T.);
#30373=ORIENTED_EDGE('',*,*,#22564,.T.);
#30374=ORIENTED_EDGE('',*,*,#22806,.F.);
#30375=ORIENTED_EDGE('',*,*,#22800,.F.);
#30376=ORIENTED_EDGE('',*,*,#22808,.T.);
#30377=ORIENTED_EDGE('',*,*,#22809,.F.);
#30378=ORIENTED_EDGE('',*,*,#22810,.T.);
#30379=ORIENTED_EDGE('',*,*,#22811,.T.);
#30380=ORIENTED_EDGE('',*,*,#22812,.F.);
#30381=ORIENTED_EDGE('',*,*,#22813,.T.);
#30382=ORIENTED_EDGE('',*,*,#22814,.F.);
#30383=ORIENTED_EDGE('',*,*,#22811,.F.);
#30384=ORIENTED_EDGE('',*,*,#22815,.T.);
#30385=ORIENTED_EDGE('',*,*,#22816,.T.);
#30386=ORIENTED_EDGE('',*,*,#22817,.F.);
#30387=ORIENTED_EDGE('',*,*,#22818,.F.);
#30388=ORIENTED_EDGE('',*,*,#22809,.T.);
#30389=ORIENTED_EDGE('',*,*,#22804,.F.);
#30390=ORIENTED_EDGE('',*,*,#22819,.F.);
#30391=ORIENTED_EDGE('',*,*,#22817,.T.);
#30392=ORIENTED_EDGE('',*,*,#22820,.T.);
#30393=ORIENTED_EDGE('',*,*,#22802,.F.);
#30394=ORIENTED_EDGE('',*,*,#22821,.F.);
#30395=ORIENTED_EDGE('',*,*,#22813,.F.);
#30396=ORIENTED_EDGE('',*,*,#22822,.T.);
#30397=ORIENTED_EDGE('',*,*,#22803,.F.);
#30398=ORIENTED_EDGE('',*,*,#22822,.F.);
#30399=ORIENTED_EDGE('',*,*,#22815,.F.);
#30400=ORIENTED_EDGE('',*,*,#22810,.F.);
#30401=ORIENTED_EDGE('',*,*,#22818,.T.);
#30402=ORIENTED_EDGE('',*,*,#22819,.T.);
#30403=ORIENTED_EDGE('',*,*,#22522,.T.);
#30404=ORIENTED_EDGE('',*,*,#22821,.T.);
#30405=ORIENTED_EDGE('',*,*,#22801,.T.);
#30406=ORIENTED_EDGE('',*,*,#22820,.F.);
#30407=ORIENTED_EDGE('',*,*,#22816,.F.);
#30408=ORIENTED_EDGE('',*,*,#22812,.T.);
#30409=ORIENTED_EDGE('',*,*,#22814,.T.);
#30410=ORIENTED_EDGE('',*,*,#22524,.F.);
#37975=CYLINDRICAL_SURFACE('',#41042,0.800100000000001);
#37976=CYLINDRICAL_SURFACE('',#41045,0.800100000000001);
#37977=CYLINDRICAL_SURFACE('',#41048,0.800100000000001);
#37978=CYLINDRICAL_SURFACE('',#41059,1.20015);
#37979=CYLINDRICAL_SURFACE('',#41061,3.556);
#37980=CYLINDRICAL_SURFACE('',#41064,1.20015);
#37981=CYLINDRICAL_SURFACE('',#41115,3.556);
#37982=CYLINDRICAL_SURFACE('',#41119,3.556);
#37983=CYLINDRICAL_SURFACE('',#41123,3.556);
#37984=CYLINDRICAL_SURFACE('',#41127,3.556);
#37985=CYLINDRICAL_SURFACE('',#41132,3.556);
#37986=CYLINDRICAL_SURFACE('',#41142,0.3556);
#37987=CYLINDRICAL_SURFACE('',#41144,0.3556);
#37988=CYLINDRICAL_SURFACE('',#41150,0.3556);
#37989=CYLINDRICAL_SURFACE('',#41152,0.3556);
#37990=CYLINDRICAL_SURFACE('',#41155,2.667);
#37991=CYLINDRICAL_SURFACE('',#41157,2.667);
#37992=CYLINDRICAL_SURFACE('',#41159,2.667);
#37993=CYLINDRICAL_SURFACE('',#41161,2.66700000000001);
#37994=CYLINDRICAL_SURFACE('',#41163,2.667);
#37995=CYLINDRICAL_SURFACE('',#41165,2.667);
#37996=CYLINDRICAL_SURFACE('',#41167,1.778);
#37997=CYLINDRICAL_SURFACE('',#41169,1.778);
#37998=CYLINDRICAL_SURFACE('',#41171,1.778);
#37999=CYLINDRICAL_SURFACE('',#41173,1.778);
#38000=CYLINDRICAL_SURFACE('',#41175,1.778);
#38001=CYLINDRICAL_SURFACE('',#41177,1.778);
#38583=ADVANCED_FACE('',(#2895),#37975,.F.);
#38584=ADVANCED_FACE('',(#2896),#37976,.F.);
#38585=ADVANCED_FACE('',(#2897),#37977,.F.);
#38586=ADVANCED_FACE('',(#2898),#31,.F.);
#38587=ADVANCED_FACE('',(#2899),#32,.F.);
#38588=ADVANCED_FACE('',(#2900),#37978,.F.);
#38589=ADVANCED_FACE('',(#2901),#37979,.T.);
#38590=ADVANCED_FACE('',(#2902),#37980,.F.);
#38591=ADVANCED_FACE('',(#2903,#226,#227,#228),#887,.T.);
#38592=ADVANCED_FACE('',(#2904),#888,.F.);
#38593=ADVANCED_FACE('',(#2905),#889,.T.);
#38594=ADVANCED_FACE('',(#2906),#890,.T.);
#38595=ADVANCED_FACE('',(#2907),#891,.F.);
#38596=ADVANCED_FACE('',(#2908),#892,.F.);
#38597=ADVANCED_FACE('',(#2909),#893,.T.);
#38598=ADVANCED_FACE('',(#2910),#894,.F.);
#38599=ADVANCED_FACE('',(#2911),#895,.T.);
#38600=ADVANCED_FACE('',(#2912),#896,.F.);
#38601=ADVANCED_FACE('',(#2913),#897,.T.);
#38602=ADVANCED_FACE('',(#2914),#898,.T.);
#38603=ADVANCED_FACE('',(#2915),#899,.F.);
#38604=ADVANCED_FACE('',(#2916,#229,#230,#231),#900,.F.);
#38605=ADVANCED_FACE('',(#2917,#232),#901,.F.);
#38606=ADVANCED_FACE('',(#2918,#233,#234,#235),#902,.T.);
#38607=ADVANCED_FACE('',(#2919),#37981,.T.);
#38608=ADVANCED_FACE('',(#2920),#903,.F.);
#38609=ADVANCED_FACE('',(#2921),#37982,.T.);
#38610=ADVANCED_FACE('',(#2922),#904,.F.);
#38611=ADVANCED_FACE('',(#2923),#37983,.T.);
#38612=ADVANCED_FACE('',(#2924),#905,.T.);
#38613=ADVANCED_FACE('',(#2925),#37984,.T.);
#38614=ADVANCED_FACE('',(#2926),#906,.T.);
#38615=ADVANCED_FACE('',(#2927),#907,.T.);
#38616=ADVANCED_FACE('',(#2928),#37985,.T.);
#38617=ADVANCED_FACE('',(#2929),#908,.T.);
#38618=ADVANCED_FACE('',(#2930,#236),#909,.F.);
#38619=ADVANCED_FACE('',(#2931),#910,.F.);
#38620=ADVANCED_FACE('',(#2932),#911,.F.);
#38621=ADVANCED_FACE('',(#2933,#237),#912,.F.);
#38622=ADVANCED_FACE('',(#2934),#2185,.T.);
#38623=ADVANCED_FACE('',(#2935),#37986,.T.);
#38624=ADVANCED_FACE('',(#2936),#37987,.T.);
#38625=ADVANCED_FACE('',(#2937),#2186,.T.);
#38626=ADVANCED_FACE('',(#2938),#2187,.T.);
#38627=ADVANCED_FACE('',(#2939),#37988,.T.);
#38628=ADVANCED_FACE('',(#2940),#37989,.T.);
#38629=ADVANCED_FACE('',(#2941),#2188,.T.);
#38630=ADVANCED_FACE('',(#2942),#37990,.T.);
#38631=ADVANCED_FACE('',(#2943),#913,.F.);
#38632=ADVANCED_FACE('',(#2944),#37991,.T.);
#38633=ADVANCED_FACE('',(#2945),#914,.T.);
#38634=ADVANCED_FACE('',(#2946),#37992,.T.);
#38635=ADVANCED_FACE('',(#2947),#915,.F.);
#38636=ADVANCED_FACE('',(#2948),#37993,.T.);
#38637=ADVANCED_FACE('',(#2949),#916,.F.);
#38638=ADVANCED_FACE('',(#2950),#37994,.T.);
#38639=ADVANCED_FACE('',(#2951),#917,.T.);
#38640=ADVANCED_FACE('',(#2952),#37995,.T.);
#38641=ADVANCED_FACE('',(#2953),#918,.T.);
#38642=ADVANCED_FACE('',(#2954),#37996,.F.);
#38643=ADVANCED_FACE('',(#2955),#919,.F.);
#38644=ADVANCED_FACE('',(#2956),#37997,.F.);
#38645=ADVANCED_FACE('',(#2957),#920,.F.);
#38646=ADVANCED_FACE('',(#2958),#37998,.F.);
#38647=ADVANCED_FACE('',(#2959),#921,.T.);
#38648=ADVANCED_FACE('',(#2960),#37999,.F.);
#38649=ADVANCED_FACE('',(#2961),#922,.F.);
#38650=ADVANCED_FACE('',(#2962),#38000,.F.);
#38651=ADVANCED_FACE('',(#2963),#923,.T.);
#38652=ADVANCED_FACE('',(#2964),#38001,.F.);
#38653=ADVANCED_FACE('',(#2965),#924,.T.);
#38654=ADVANCED_FACE('',(#2966),#925,.F.);
#38655=ADVANCED_FACE('',(#2967),#926,.F.);
#38656=ADVANCED_FACE('',(#2968),#927,.T.);
#38657=ADVANCED_FACE('',(#2969),#928,.F.);
#38658=ADVANCED_FACE('',(#2970),#929,.T.);
#38659=ADVANCED_FACE('',(#2971),#930,.F.);
#38660=ADVANCED_FACE('',(#2972),#931,.T.);
#38661=ADVANCED_FACE('',(#2973),#932,.T.);
#38662=ADVANCED_FACE('',(#2974),#933,.F.);
#38663=ADVANCED_FACE('',(#2975,#238),#934,.F.);
#38664=ADVANCED_FACE('',(#2976),#935,.F.);
#38665=ADVANCED_FACE('',(#2977),#936,.T.);
#38666=ADVANCED_FACE('',(#2978),#937,.F.);
#38667=ADVANCED_FACE('',(#2979),#938,.T.);
#38668=ADVANCED_FACE('',(#2980),#939,.T.);
#38669=ADVANCED_FACE('',(#2981),#940,.F.);
#38670=ADVANCED_FACE('',(#2982),#941,.F.);
#38671=ADVANCED_FACE('',(#2983),#942,.F.);
#38672=ADVANCED_FACE('',(#2984,#239),#943,.T.);
#38673=ADVANCED_FACE('',(#2985),#944,.F.);
#38674=ADVANCED_FACE('',(#2986,#240),#945,.F.);
#38675=ADVANCED_FACE('',(#2987),#946,.T.);
#38676=ADVANCED_FACE('',(#2988),#947,.F.);
#38677=ADVANCED_FACE('',(#2989),#948,.T.);
#38678=ADVANCED_FACE('',(#2990),#949,.F.);
#38679=ADVANCED_FACE('',(#2991,#241),#950,.T.);
#38680=ADVANCED_FACE('',(#2992),#951,.F.);
#38681=ADVANCED_FACE('',(#2993),#952,.T.);
#38682=ADVANCED_FACE('',(#2994),#953,.F.);
#38683=ADVANCED_FACE('',(#2995),#954,.T.);
#38684=ADVANCED_FACE('',(#2996),#955,.T.);
#38685=ADVANCED_FACE('',(#2997,#242),#956,.T.);
#38686=ADVANCED_FACE('',(#2998,#243),#957,.F.);
#38687=ADVANCED_FACE('',(#2999,#244),#958,.F.);
#38688=ADVANCED_FACE('',(#3000),#959,.T.);
#38689=ADVANCED_FACE('',(#3001),#960,.F.);
#38690=ADVANCED_FACE('',(#3002),#961,.T.);
#38691=ADVANCED_FACE('',(#3003),#962,.F.);
#38692=ADVANCED_FACE('',(#3004),#963,.T.);
#38693=ADVANCED_FACE('',(#3005),#964,.T.);
#38694=ADVANCED_FACE('',(#3006),#965,.F.);
#38695=ADVANCED_FACE('',(#3007),#966,.F.);
#38696=ADVANCED_FACE('',(#3008),#967,.F.);
#38697=ADVANCED_FACE('',(#3009,#245),#968,.F.);
#38698=ADVANCED_FACE('',(#3010,#246),#969,.T.);
#39934=CLOSED_SHELL('',(#38583,#38584,#38585,#38586,#38587,#38588,#38589,
#38590,#38591,#38592,#38593,#38594,#38595,#38596,#38597,#38598,#38599,#38600,
#38601,#38602,#38603,#38604,#38605,#38606,#38607,#38608,#38609,#38610,#38611,
#38612,#38613,#38614,#38615,#38616,#38617,#38618,#38619,#38620,#38621,#38622,
#38623,#38624,#38625,#38626,#38627,#38628,#38629,#38630,#38631,#38632,#38633,
#38634,#38635,#38636,#38637,#38638,#38639,#38640,#38641,#38642,#38643,#38644,
#38645,#38646,#38647,#38648,#38649,#38650,#38651,#38652,#38653,#38654,#38655,
#38656,#38657,#38658,#38659,#38660,#38661,#38662,#38663,#38664,#38665,#38666,
#38667,#38668,#38669,#38670,#38671,#38672,#38673,#38674,#38675,#38676,#38677,
#38678,#38679,#38680,#38681,#38682,#38683,#38684,#38685,#38686,#38687,#38688,
#38689,#38690,#38691,#38692,#38693,#38694,#38695,#38696,#38697,#38698));
#41041=AXIS2_PLACEMENT_3D('',#57363,#45666,#45667);
#41042=AXIS2_PLACEMENT_3D('',#57364,#45668,#45669);
#41043=AXIS2_PLACEMENT_3D('',#57366,#45670,#45671);
#41044=AXIS2_PLACEMENT_3D('',#57369,#45673,#45674);
#41045=AXIS2_PLACEMENT_3D('',#57370,#45675,#45676);
#41046=AXIS2_PLACEMENT_3D('',#57372,#45677,#45678);
#41047=AXIS2_PLACEMENT_3D('',#57375,#45680,#45681);
#41048=AXIS2_PLACEMENT_3D('',#57376,#45682,#45683);
#41049=AXIS2_PLACEMENT_3D('',#57378,#45684,#45685);
#41050=AXIS2_PLACEMENT_3D('',#57381,#45687,#45688);
#41051=AXIS2_PLACEMENT_3D('',#57382,#45689,#45690);
#41052=AXIS2_PLACEMENT_3D('',#57385,#45691,#45692);
#41053=AXIS2_PLACEMENT_3D('',#57386,#45693,#45694);
#41054=AXIS2_PLACEMENT_3D('',#57389,#45696,#45697);
#41055=AXIS2_PLACEMENT_3D('',#57390,#45698,#45699);
#41056=AXIS2_PLACEMENT_3D('',#57393,#45700,#45701);
#41057=AXIS2_PLACEMENT_3D('',#57394,#45702,#45703);
#41058=AXIS2_PLACEMENT_3D('',#57397,#45705,#45706);
#41059=AXIS2_PLACEMENT_3D('',#57398,#45707,#45708);
#41060=AXIS2_PLACEMENT_3D('',#57401,#45710,#45711);
#41061=AXIS2_PLACEMENT_3D('',#57402,#45712,#45713);
#41062=AXIS2_PLACEMENT_3D('',#57405,#45714,#45715);
#41063=AXIS2_PLACEMENT_3D('',#57409,#45717,#45718);
#41064=AXIS2_PLACEMENT_3D('',#57411,#45720,#45721);
#41065=AXIS2_PLACEMENT_3D('',#57414,#45723,#45724);
#41066=AXIS2_PLACEMENT_3D('',#57415,#45725,#45726);
#41067=AXIS2_PLACEMENT_3D('',#57418,#45727,#45728);
#41068=AXIS2_PLACEMENT_3D('',#57422,#45730,#45731);
#41069=AXIS2_PLACEMENT_3D('',#57426,#45733,#45734);
#41070=AXIS2_PLACEMENT_3D('',#57430,#45736,#45737);
#41071=AXIS2_PLACEMENT_3D('',#57434,#45739,#45740);
#41072=AXIS2_PLACEMENT_3D('',#57438,#45742,#45743);
#41073=AXIS2_PLACEMENT_3D('',#57464,#45757,#45758);
#41074=AXIS2_PLACEMENT_3D('',#57473,#45763,#45764);
#41075=AXIS2_PLACEMENT_3D('',#57483,#45770,#45771);
#41076=AXIS2_PLACEMENT_3D('',#57493,#45777,#45778);
#41077=AXIS2_PLACEMENT_3D('',#57496,#45781,#45782);
#41078=AXIS2_PLACEMENT_3D('',#57509,#45789,#45790);
#41079=AXIS2_PLACEMENT_3D('',#57515,#45794,#45795);
#41080=AXIS2_PLACEMENT_3D('',#57525,#45801,#45802);
#41081=AXIS2_PLACEMENT_3D('',#57528,#45805,#45806);
#41082=AXIS2_PLACEMENT_3D('',#57537,#45811,#45812);
#41083=AXIS2_PLACEMENT_3D('',#57547,#45818,#45819);
#41084=AXIS2_PLACEMENT_3D('',#57557,#45825,#45826);
#41085=AXIS2_PLACEMENT_3D('',#57560,#45829,#45830);
#41086=AXIS2_PLACEMENT_3D('',#57563,#45831,#45832);
#41087=AXIS2_PLACEMENT_3D('',#57567,#45834,#45835);
#41088=AXIS2_PLACEMENT_3D('',#57571,#45837,#45838);
#41089=AXIS2_PLACEMENT_3D('',#57575,#45840,#45841);
#41090=AXIS2_PLACEMENT_3D('',#57579,#45843,#45844);
#41091=AXIS2_PLACEMENT_3D('',#57583,#45846,#45847);
#41092=AXIS2_PLACEMENT_3D('',#57588,#45852,#45853);
#41093=AXIS2_PLACEMENT_3D('',#57593,#45855,#45856);
#41094=AXIS2_PLACEMENT_3D('',#57597,#45858,#45859);
#41095=AXIS2_PLACEMENT_3D('',#57601,#45861,#45862);
#41096=AXIS2_PLACEMENT_3D('',#57604,#45864,#45865);
#41097=AXIS2_PLACEMENT_3D('',#57607,#45866,#45867);
#41098=AXIS2_PLACEMENT_3D('',#57611,#45869,#45870);
#41099=AXIS2_PLACEMENT_3D('',#57615,#45872,#45873);
#41100=AXIS2_PLACEMENT_3D('',#57619,#45875,#45876);
#41101=AXIS2_PLACEMENT_3D('',#57623,#45878,#45879);
#41102=AXIS2_PLACEMENT_3D('',#57627,#45881,#45882);
#41103=AXIS2_PLACEMENT_3D('',#57629,#45884,#45885);
#41104=AXIS2_PLACEMENT_3D('',#57633,#45887,#45888);
#41105=AXIS2_PLACEMENT_3D('',#57637,#45890,#45891);
#41106=AXIS2_PLACEMENT_3D('',#57641,#45893,#45894);
#41107=AXIS2_PLACEMENT_3D('',#57645,#45896,#45897);
#41108=AXIS2_PLACEMENT_3D('',#57649,#45899,#45900);
#41109=AXIS2_PLACEMENT_3D('',#57655,#45903,#45904);
#41110=AXIS2_PLACEMENT_3D('',#57659,#45906,#45907);
#41111=AXIS2_PLACEMENT_3D('',#57663,#45909,#45910);
#41112=AXIS2_PLACEMENT_3D('',#57667,#45912,#45913);
#41113=AXIS2_PLACEMENT_3D('',#57671,#45915,#45916);
#41114=AXIS2_PLACEMENT_3D('',#57674,#45918,#45919);
#41115=AXIS2_PLACEMENT_3D('',#57675,#45920,#45921);
#41116=AXIS2_PLACEMENT_3D('',#57680,#45923,#45924);
#41117=AXIS2_PLACEMENT_3D('',#57684,#45927,#45928);
#41118=AXIS2_PLACEMENT_3D('',#57685,#45929,#45930);
#41119=AXIS2_PLACEMENT_3D('',#57691,#45934,#45935);
#41120=AXIS2_PLACEMENT_3D('',#57696,#45937,#45938);
#41121=AXIS2_PLACEMENT_3D('',#57700,#45941,#45942);
#41122=AXIS2_PLACEMENT_3D('',#57701,#45943,#45944);
#41123=AXIS2_PLACEMENT_3D('',#57707,#45948,#45949);
#41124=AXIS2_PLACEMENT_3D('',#57710,#45951,#45952);
#41125=AXIS2_PLACEMENT_3D('',#57712,#45953,#45954);
#41126=AXIS2_PLACEMENT_3D('',#57714,#45956,#45957);
#41127=AXIS2_PLACEMENT_3D('',#57716,#45959,#45960);
#41128=AXIS2_PLACEMENT_3D('',#57719,#45962,#45963);
#41129=AXIS2_PLACEMENT_3D('',#57721,#45964,#45965);
#41130=AXIS2_PLACEMENT_3D('',#57723,#45967,#45968);
#41131=AXIS2_PLACEMENT_3D('',#57725,#45970,#45971);
#41132=AXIS2_PLACEMENT_3D('',#57729,#45974,#45975);
#41133=AXIS2_PLACEMENT_3D('',#57732,#45977,#45978);
#41134=AXIS2_PLACEMENT_3D('',#57733,#45979,#45980);
#41135=AXIS2_PLACEMENT_3D('',#57735,#45982,#45983);
#41136=AXIS2_PLACEMENT_3D('',#57736,#45984,#45985);
#41137=AXIS2_PLACEMENT_3D('',#57738,#45987,#45988);
#41138=AXIS2_PLACEMENT_3D('',#57740,#45990,#45991);
#41139=AXIS2_PLACEMENT_3D('',#57741,#45992,#45993);
#41140=AXIS2_PLACEMENT_3D('',#57742,#45994,#45995);
#41141=AXIS2_PLACEMENT_3D('',#57743,#45996,#45997);
#41142=AXIS2_PLACEMENT_3D('',#57744,#45998,#45999);
#41143=AXIS2_PLACEMENT_3D('',#57745,#46000,#46001);
#41144=AXIS2_PLACEMENT_3D('',#57746,#46002,#46003);
#41145=AXIS2_PLACEMENT_3D('',#57747,#46004,#46005);
#41146=AXIS2_PLACEMENT_3D('',#57748,#46006,#46007);
#41147=AXIS2_PLACEMENT_3D('',#57749,#46008,#46009);
#41148=AXIS2_PLACEMENT_3D('',#57750,#46010,#46011);
#41149=AXIS2_PLACEMENT_3D('',#57751,#46012,#46013);
#41150=AXIS2_PLACEMENT_3D('',#57752,#46014,#46015);
#41151=AXIS2_PLACEMENT_3D('',#57753,#46016,#46017);
#41152=AXIS2_PLACEMENT_3D('',#57754,#46018,#46019);
#41153=AXIS2_PLACEMENT_3D('',#57755,#46020,#46021);
#41154=AXIS2_PLACEMENT_3D('',#57756,#46022,#46023);
#41155=AXIS2_PLACEMENT_3D('',#57757,#46024,#46025);
#41156=AXIS2_PLACEMENT_3D('',#57760,#46028,#46029);
#41157=AXIS2_PLACEMENT_3D('',#57762,#46031,#46032);
#41158=AXIS2_PLACEMENT_3D('',#57764,#46034,#46035);
#41159=AXIS2_PLACEMENT_3D('',#57766,#46037,#46038);
#41160=AXIS2_PLACEMENT_3D('',#57768,#46040,#46041);
#41161=AXIS2_PLACEMENT_3D('',#57770,#46043,#46044);
#41162=AXIS2_PLACEMENT_3D('',#57772,#46046,#46047);
#41163=AXIS2_PLACEMENT_3D('',#57774,#46049,#46050);
#41164=AXIS2_PLACEMENT_3D('',#57776,#46052,#46053);
#41165=AXIS2_PLACEMENT_3D('',#57778,#46055,#46056);
#41166=AXIS2_PLACEMENT_3D('',#57780,#46058,#46059);
#41167=AXIS2_PLACEMENT_3D('',#57781,#46060,#46061);
#41168=AXIS2_PLACEMENT_3D('',#57784,#46064,#46065);
#41169=AXIS2_PLACEMENT_3D('',#57786,#46067,#46068);
#41170=AXIS2_PLACEMENT_3D('',#57788,#46070,#46071);
#41171=AXIS2_PLACEMENT_3D('',#57790,#46073,#46074);
#41172=AXIS2_PLACEMENT_3D('',#57792,#46076,#46077);
#41173=AXIS2_PLACEMENT_3D('',#57794,#46079,#46080);
#41174=AXIS2_PLACEMENT_3D('',#57796,#46082,#46083);
#41175=AXIS2_PLACEMENT_3D('',#57798,#46085,#46086);
#41176=AXIS2_PLACEMENT_3D('',#57800,#46088,#46089);
#41177=AXIS2_PLACEMENT_3D('',#57802,#46091,#46092);
#41178=AXIS2_PLACEMENT_3D('',#57804,#46094,#46095);
#41179=AXIS2_PLACEMENT_3D('',#57805,#46096,#46097);
#41180=AXIS2_PLACEMENT_3D('',#57807,#46099,#46100);
#41181=AXIS2_PLACEMENT_3D('',#57809,#46102,#46103);
#41182=AXIS2_PLACEMENT_3D('',#57811,#46105,#46106);
#41183=AXIS2_PLACEMENT_3D('',#57812,#46107,#46108);
#41184=AXIS2_PLACEMENT_3D('',#57813,#46109,#46110);
#41185=AXIS2_PLACEMENT_3D('',#57814,#46111,#46112);
#41186=AXIS2_PLACEMENT_3D('',#57815,#46113,#46114);
#41187=AXIS2_PLACEMENT_3D('',#57816,#46115,#46116);
#41188=AXIS2_PLACEMENT_3D('',#57817,#46117,#46118);
#41189=AXIS2_PLACEMENT_3D('',#57834,#46127,#46128);
#41190=AXIS2_PLACEMENT_3D('',#57837,#46131,#46132);
#41191=AXIS2_PLACEMENT_3D('',#57839,#46134,#46135);
#41192=AXIS2_PLACEMENT_3D('',#57841,#46137,#46138);
#41193=AXIS2_PLACEMENT_3D('',#57842,#46139,#46140);
#41194=AXIS2_PLACEMENT_3D('',#57851,#46145,#46146);
#41195=AXIS2_PLACEMENT_3D('',#57857,#46150,#46151);
#41196=AXIS2_PLACEMENT_3D('',#57863,#46155,#46156);
#41197=AXIS2_PLACEMENT_3D('',#57866,#46159,#46160);
#41198=AXIS2_PLACEMENT_3D('',#57868,#46162,#46163);
#41199=AXIS2_PLACEMENT_3D('',#57870,#46165,#46166);
#41200=AXIS2_PLACEMENT_3D('',#57871,#46167,#46168);
#41201=AXIS2_PLACEMENT_3D('',#57877,#46172,#46173);
#41202=AXIS2_PLACEMENT_3D('',#57881,#46176,#46177);
#41203=AXIS2_PLACEMENT_3D('',#57885,#46180,#46181);
#41204=AXIS2_PLACEMENT_3D('',#57887,#46183,#46184);
#41205=AXIS2_PLACEMENT_3D('',#57896,#46189,#46190);
#41206=AXIS2_PLACEMENT_3D('',#57905,#46195,#46196);
#41207=AXIS2_PLACEMENT_3D('',#57911,#46200,#46201);
#41208=AXIS2_PLACEMENT_3D('',#57917,#46205,#46206);
#41209=AXIS2_PLACEMENT_3D('',#57920,#46209,#46210);
#41210=AXIS2_PLACEMENT_3D('',#57923,#46213,#46214);
#41211=AXIS2_PLACEMENT_3D('',#57924,#46215,#46216);
#41212=AXIS2_PLACEMENT_3D('',#57925,#46217,#46218);
#41213=AXIS2_PLACEMENT_3D('',#57942,#46227,#46228);
#41214=AXIS2_PLACEMENT_3D('',#57945,#46231,#46232);
#41215=AXIS2_PLACEMENT_3D('',#57947,#46234,#46235);
#41216=AXIS2_PLACEMENT_3D('',#57949,#46237,#46238);
#41217=AXIS2_PLACEMENT_3D('',#57950,#46239,#46240);
#41218=AXIS2_PLACEMENT_3D('',#57959,#46245,#46246);
#41219=AXIS2_PLACEMENT_3D('',#57965,#46250,#46251);
#41220=AXIS2_PLACEMENT_3D('',#57971,#46255,#46256);
#41221=AXIS2_PLACEMENT_3D('',#57974,#46259,#46260);
#41222=AXIS2_PLACEMENT_3D('',#57977,#46263,#46264);
#41223=AXIS2_PLACEMENT_3D('',#57978,#46265,#46266);
#45666=DIRECTION('axis',(0.,0.,1.));
#45667=DIRECTION('refdir',(1.,0.,0.));
#45668=DIRECTION('center_axis',(1.,0.,0.));
#45669=DIRECTION('ref_axis',(0.,0.,-1.));
#45670=DIRECTION('center_axis',(1.,0.,0.));
#45671=DIRECTION('ref_axis',(0.,0.,-1.));
#45672=DIRECTION('',(1.,0.,0.));
#45673=DIRECTION('center_axis',(1.,0.,0.));
#45674=DIRECTION('ref_axis',(0.,0.,-1.));
#45675=DIRECTION('center_axis',(1.,0.,0.));
#45676=DIRECTION('ref_axis',(0.,0.,-1.));
#45677=DIRECTION('center_axis',(-1.,0.,0.));
#45678=DIRECTION('ref_axis',(0.,0.,1.));
#45679=DIRECTION('',(1.,0.,0.));
#45680=DIRECTION('center_axis',(1.,0.,0.));
#45681=DIRECTION('ref_axis',(0.,0.,-1.));
#45682=DIRECTION('center_axis',(1.,0.,0.));
#45683=DIRECTION('ref_axis',(0.,0.,-1.));
#45684=DIRECTION('center_axis',(-1.,2.06958181338202E-16,0.));
#45685=DIRECTION('ref_axis',(2.06958181338202E-16,1.,0.));
#45686=DIRECTION('',(1.,0.,0.));
#45687=DIRECTION('center_axis',(-1.,-1.29348863336376E-16,0.));
#45688=DIRECTION('ref_axis',(-1.29348863336376E-16,1.,0.));
#45689=DIRECTION('center_axis',(0.,0.,1.));
#45690=DIRECTION('ref_axis',(1.,0.,0.));
#45691=DIRECTION('center_axis',(0.,0.,1.));
#45692=DIRECTION('ref_axis',(-1.,0.,0.));
#45693=DIRECTION('center_axis',(0.,0.,1.));
#45694=DIRECTION('ref_axis',(-1.,0.,0.));
#45695=DIRECTION('',(-0.656059028990511,-8.0344058990495E-17,0.754709580222769));
#45696=DIRECTION('center_axis',(0.,0.,-1.));
#45697=DIRECTION('ref_axis',(-1.,0.,0.));
#45698=DIRECTION('center_axis',(0.,0.,1.));
#45699=DIRECTION('ref_axis',(1.,0.,0.));
#45700=DIRECTION('center_axis',(0.,0.,1.));
#45701=DIRECTION('ref_axis',(-1.,0.,0.));
#45702=DIRECTION('center_axis',(0.,0.,1.));
#45703=DIRECTION('ref_axis',(-1.,0.,0.));
#45704=DIRECTION('',(-0.656059028990511,-8.0344058990495E-17,0.754709580222769));
#45705=DIRECTION('center_axis',(0.,0.,-1.));
#45706=DIRECTION('ref_axis',(-1.,0.,0.));
#45707=DIRECTION('center_axis',(0.,0.,-1.));
#45708=DIRECTION('ref_axis',(-1.,0.,0.));
#45709=DIRECTION('',(0.,0.,-1.));
#45710=DIRECTION('center_axis',(0.,0.,-1.));
#45711=DIRECTION('ref_axis',(-1.,0.,0.));
#45712=DIRECTION('center_axis',(0.,0.,-1.));
#45713=DIRECTION('ref_axis',(-1.,0.,0.));
#45714=DIRECTION('center_axis',(0.,0.,1.));
#45715=DIRECTION('ref_axis',(1.,0.,0.));
#45716=DIRECTION('',(0.,0.,-1.));
#45717=DIRECTION('center_axis',(0.,0.,1.));
#45718=DIRECTION('ref_axis',(1.,0.,0.));
#45719=DIRECTION('',(0.,0.,-1.));
#45720=DIRECTION('center_axis',(0.,0.,-1.));
#45721=DIRECTION('ref_axis',(-1.,0.,0.));
#45722=DIRECTION('',(0.,0.,-1.));
#45723=DIRECTION('center_axis',(0.,0.,-1.));
#45724=DIRECTION('ref_axis',(-1.,0.,0.));
#45725=DIRECTION('center_axis',(0.,0.,-1.));
#45726=DIRECTION('ref_axis',(-1.,0.,0.));
#45727=DIRECTION('center_axis',(0.,0.,-1.));
#45728=DIRECTION('ref_axis',(-1.,0.,0.));
#45729=DIRECTION('',(1.,0.,0.));
#45730=DIRECTION('center_axis',(0.,0.,1.));
#45731=DIRECTION('ref_axis',(1.,0.,0.));
#45732=DIRECTION('',(-2.33197918015441E-16,1.,0.));
#45733=DIRECTION('center_axis',(0.,0.,-1.));
#45734=DIRECTION('ref_axis',(-1.,0.,0.));
#45735=DIRECTION('',(-0.707106781186543,-0.707106781186552,0.));
#45736=DIRECTION('center_axis',(0.,0.,1.));
#45737=DIRECTION('ref_axis',(1.,0.,0.));
#45738=DIRECTION('',(-1.,3.20838317005448E-16,0.));
#45739=DIRECTION('center_axis',(0.,0.,-1.));
#45740=DIRECTION('ref_axis',(-1.,0.,0.));
#45741=DIRECTION('',(0.707106781186544,-0.707106781186551,0.));
#45742=DIRECTION('center_axis',(0.,0.,1.));
#45743=DIRECTION('ref_axis',(1.,0.,0.));
#45744=DIRECTION('',(2.33197918015441E-16,-1.,0.));
#45745=DIRECTION('',(6.96899998383741E-17,1.,0.));
#45746=DIRECTION('',(1.,0.,0.));
#45747=DIRECTION('',(1.39379999676748E-16,-1.,0.));
#45748=DIRECTION('',(-1.,0.,0.));
#45749=DIRECTION('',(-1.39379999676748E-16,1.,0.));
#45750=DIRECTION('',(1.,6.44303772090628E-16,0.));
#45751=DIRECTION('',(5.57519998706993E-16,-1.,0.));
#45752=DIRECTION('',(-1.,0.,0.));
#45753=DIRECTION('',(1.,0.,0.));
#45754=DIRECTION('',(-2.78759999353496E-16,-1.,0.));
#45755=DIRECTION('',(-1.,-6.44303772090628E-16,0.));
#45756=DIRECTION('',(2.78759999353496E-16,1.,0.));
#45757=DIRECTION('center_axis',(1.,1.55218636003651E-16,0.));
#45758=DIRECTION('ref_axis',(-1.55218636003651E-16,1.,0.));
#45759=DIRECTION('',(1.55218636003651E-16,-1.,4.48409752679708E-16));
#45760=DIRECTION('',(0.,0.,-1.));
#45761=DIRECTION('',(1.55218636003651E-16,-1.,0.));
#45762=DIRECTION('',(0.,0.,-1.));
#45763=DIRECTION('center_axis',(0.,-1.,0.));
#45764=DIRECTION('ref_axis',(0.,0.,-1.));
#45765=DIRECTION('',(0.327110329510081,0.,-0.94498615456937));
#45766=DIRECTION('',(-1.,0.,0.));
#45767=DIRECTION('',(-0.327110329510081,0.,-0.94498615456937));
#45768=DIRECTION('',(-1.,0.,0.));
#45769=DIRECTION('',(0.,0.,-1.));
#45770=DIRECTION('center_axis',(0.,1.,0.));
#45771=DIRECTION('ref_axis',(0.,0.,1.));
#45772=DIRECTION('',(0.327110329510081,0.,-0.94498615456937));
#45773=DIRECTION('',(0.,0.,-1.));
#45774=DIRECTION('',(1.,0.,0.));
#45775=DIRECTION('',(-0.327110329510081,0.,-0.94498615456937));
#45776=DIRECTION('',(1.,0.,0.));
#45777=DIRECTION('center_axis',(0.,0.,-1.));
#45778=DIRECTION('ref_axis',(-1.,0.,0.));
#45779=DIRECTION('',(0.,1.,0.));
#45780=DIRECTION('',(0.,1.,0.));
#45781=DIRECTION('center_axis',(0.,-1.,0.));
#45782=DIRECTION('ref_axis',(0.,0.,-1.));
#45783=DIRECTION('',(-0.216439613938104,0.,-0.976296007119933));
#45784=DIRECTION('',(-1.,0.,0.));
#45785=DIRECTION('',(0.216439613938104,0.,-0.976296007119933));
#45786=DIRECTION('',(0.,0.,-1.));
#45787=DIRECTION('',(-1.,0.,0.));
#45788=DIRECTION('',(0.,0.,-1.));
#45789=DIRECTION('center_axis',(-1.,2.06958181338202E-16,0.));
#45790=DIRECTION('ref_axis',(-2.06958181338202E-16,-1.,0.));
#45791=DIRECTION('',(0.,0.,-1.));
#45792=DIRECTION('',(2.06958181338202E-16,1.,9.33528028464658E-16));
#45793=DIRECTION('',(2.06958181338202E-16,1.,0.));
#45794=DIRECTION('center_axis',(0.,1.,0.));
#45795=DIRECTION('ref_axis',(0.,0.,1.));
#45796=DIRECTION('',(-0.216439613938104,0.,-0.976296007119933));
#45797=DIRECTION('',(1.,0.,0.));
#45798=DIRECTION('',(0.,0.,-1.));
#45799=DIRECTION('',(0.216439613938104,0.,-0.976296007119933));
#45800=DIRECTION('',(1.,0.,0.));
#45801=DIRECTION('center_axis',(0.,0.,1.));
#45802=DIRECTION('ref_axis',(1.,0.,0.));
#45803=DIRECTION('',(0.,-1.,0.));
#45804=DIRECTION('',(0.,-1.,0.));
#45805=DIRECTION('center_axis',(1.,6.20874544014605E-16,0.));
#45806=DIRECTION('ref_axis',(-6.20874544014605E-16,1.,0.));
#45807=DIRECTION('',(6.20874544014605E-16,-1.,2.80058408539398E-15));
#45808=DIRECTION('',(0.,0.,-1.));
#45809=DIRECTION('',(6.20874544014605E-16,-1.,0.));
#45810=DIRECTION('',(0.,0.,-1.));
#45811=DIRECTION('center_axis',(0.,-1.,0.));
#45812=DIRECTION('ref_axis',(0.,0.,-1.));
#45813=DIRECTION('',(-1.,0.,0.));
#45814=DIRECTION('',(-0.216439613938103,0.,-0.976296007119933));
#45815=DIRECTION('',(-1.,0.,0.));
#45816=DIRECTION('',(0.,0.,-1.));
#45817=DIRECTION('',(0.216439613938103,0.,-0.976296007119933));
#45818=DIRECTION('center_axis',(0.,1.,0.));
#45819=DIRECTION('ref_axis',(0.,0.,1.));
#45820=DIRECTION('',(0.216439613938103,0.,0.976296007119933));
#45821=DIRECTION('',(1.,0.,0.));
#45822=DIRECTION('',(-0.216439613938103,0.,0.976296007119933));
#45823=DIRECTION('',(0.,0.,-1.));
#45824=DIRECTION('',(1.,0.,0.));
#45825=DIRECTION('center_axis',(0.,0.,-1.));
#45826=DIRECTION('ref_axis',(-1.,0.,0.));
#45827=DIRECTION('',(0.,1.,0.));
#45828=DIRECTION('',(0.,1.,0.));
#45829=DIRECTION('center_axis',(0.,0.,-1.));
#45830=DIRECTION('ref_axis',(-1.,0.,0.));
#45831=DIRECTION('center_axis',(0.,0.,-1.));
#45832=DIRECTION('ref_axis',(-1.,0.,0.));
#45833=DIRECTION('',(-1.,0.,0.));
#45834=DIRECTION('center_axis',(0.,0.,1.));
#45835=DIRECTION('ref_axis',(1.,0.,0.));
#45836=DIRECTION('',(-0.707106781186544,-0.707106781186551,0.));
#45837=DIRECTION('center_axis',(0.,0.,-1.));
#45838=DIRECTION('ref_axis',(-1.,0.,0.));
#45839=DIRECTION('',(0.,1.,0.));
#45840=DIRECTION('center_axis',(0.,0.,1.));
#45841=DIRECTION('ref_axis',(1.,0.,0.));
#45842=DIRECTION('',(1.,0.,0.));
#45843=DIRECTION('center_axis',(0.,0.,-1.));
#45844=DIRECTION('ref_axis',(-1.,0.,0.));
#45845=DIRECTION('',(0.,-1.,0.));
#45846=DIRECTION('center_axis',(0.,0.,1.));
#45847=DIRECTION('ref_axis',(1.,0.,0.));
#45848=DIRECTION('',(0.707106781186544,-0.707106781186551,0.));
#45849=DIRECTION('',(-2.06958181338202E-16,1.,0.));
#45850=DIRECTION('',(-6.20874544014605E-16,-1.,0.));
#45851=DIRECTION('',(0.,1.,0.));
#45852=DIRECTION('center_axis',(0.,0.,-1.));
#45853=DIRECTION('ref_axis',(-1.,0.,0.));
#45854=DIRECTION('',(0.,-1.,0.));
#45855=DIRECTION('center_axis',(0.,0.,1.));
#45856=DIRECTION('ref_axis',(-1.,0.,0.));
#45857=DIRECTION('',(1.,-1.52617206349959E-16,0.));
#45858=DIRECTION('center_axis',(0.,0.,1.));
#45859=DIRECTION('ref_axis',(-1.,0.,0.));
#45860=DIRECTION('',(0.,1.,0.));
#45861=DIRECTION('center_axis',(0.,0.,1.));
#45862=DIRECTION('ref_axis',(-1.,1.89711666226685E-15,0.));
#45863=DIRECTION('',(-1.,0.,0.));
#45864=DIRECTION('center_axis',(0.,0.,1.));
#45865=DIRECTION('ref_axis',(-1.,2.38494666113547E-14,0.));
#45866=DIRECTION('center_axis',(0.,0.,-1.));
#45867=DIRECTION('ref_axis',(-1.,0.,0.));
#45868=DIRECTION('',(0.707106781186544,-0.707106781186551,0.));
#45869=DIRECTION('center_axis',(0.,0.,1.));
#45870=DIRECTION('ref_axis',(1.,0.,0.));
#45871=DIRECTION('',(0.,-1.,0.));
#45872=DIRECTION('center_axis',(0.,0.,-1.));
#45873=DIRECTION('ref_axis',(-1.,0.,0.));
#45874=DIRECTION('',(1.,0.,0.));
#45875=DIRECTION('center_axis',(0.,0.,1.));
#45876=DIRECTION('ref_axis',(1.,0.,0.));
#45877=DIRECTION('',(0.,1.,0.));
#45878=DIRECTION('center_axis',(0.,0.,-1.));
#45879=DIRECTION('ref_axis',(-1.,0.,0.));
#45880=DIRECTION('',(-0.707106781186544,-0.707106781186551,0.));
#45881=DIRECTION('center_axis',(0.,0.,1.));
#45882=DIRECTION('ref_axis',(1.,0.,0.));
#45883=DIRECTION('',(-1.,0.,0.));
#45884=DIRECTION('center_axis',(0.,0.,-1.));
#45885=DIRECTION('ref_axis',(-1.,0.,0.));
#45886=DIRECTION('',(-0.826053778523829,-0.563591301375832,0.));
#45887=DIRECTION('center_axis',(0.,0.,-1.));
#45888=DIRECTION('ref_axis',(-1.,0.,0.));
#45889=DIRECTION('',(1.,0.,0.));
#45890=DIRECTION('center_axis',(0.,0.,1.));
#45891=DIRECTION('ref_axis',(1.,0.,0.));
#45892=DIRECTION('',(0.826053778523829,-0.563591301375832,0.));
#45893=DIRECTION('center_axis',(0.,0.,-1.));
#45894=DIRECTION('ref_axis',(-1.,0.,0.));
#45895=DIRECTION('',(-0.82605377852383,-0.563591301375832,0.));
#45896=DIRECTION('center_axis',(0.,0.,-1.));
#45897=DIRECTION('ref_axis',(-1.,0.,0.));
#45898=DIRECTION('',(-1.,1.52617206349959E-16,0.));
#45899=DIRECTION('center_axis',(0.,0.,-1.));
#45900=DIRECTION('ref_axis',(-1.,0.,0.));
#45901=DIRECTION('',(0.82605377852383,-0.563591301375832,0.));
#45902=DIRECTION('',(1.,0.,0.));
#45903=DIRECTION('center_axis',(0.,0.,-1.));
#45904=DIRECTION('ref_axis',(-1.,0.,0.));
#45905=DIRECTION('',(2.33197918015441E-16,-1.,0.));
#45906=DIRECTION('center_axis',(0.,0.,1.));
#45907=DIRECTION('ref_axis',(1.,0.,0.));
#45908=DIRECTION('',(0.707106781186544,-0.707106781186551,0.));
#45909=DIRECTION('center_axis',(0.,0.,-1.));
#45910=DIRECTION('ref_axis',(-1.,0.,0.));
#45911=DIRECTION('',(-1.,3.20838317005448E-16,0.));
#45912=DIRECTION('center_axis',(0.,0.,1.));
#45913=DIRECTION('ref_axis',(1.,0.,0.));
#45914=DIRECTION('',(-0.707106781186543,-0.707106781186552,0.));
#45915=DIRECTION('center_axis',(0.,0.,-1.));
#45916=DIRECTION('ref_axis',(-1.,0.,0.));
#45917=DIRECTION('',(-2.33197918015441E-16,1.,0.));
#45918=DIRECTION('center_axis',(0.,0.,1.));
#45919=DIRECTION('ref_axis',(1.,0.,0.));
#45920=DIRECTION('center_axis',(0.,0.,-1.));
#45921=DIRECTION('ref_axis',(-1.,0.,0.));
#45922=DIRECTION('',(0.,0.,-1.));
#45923=DIRECTION('center_axis',(0.,0.,-1.));
#45924=DIRECTION('ref_axis',(-1.,0.,0.));
#45925=DIRECTION('',(0.,0.,-1.));
#45926=DIRECTION('',(0.,0.,-1.));
#45927=DIRECTION('center_axis',(0.,0.,-1.));
#45928=DIRECTION('ref_axis',(-1.,0.,0.));
#45929=DIRECTION('center_axis',(1.,0.,0.));
#45930=DIRECTION('ref_axis',(0.,0.,-1.));
#45931=DIRECTION('',(0.,0.,-1.));
#45932=DIRECTION('',(0.,1.,0.));
#45933=DIRECTION('',(0.,-1.,0.));
#45934=DIRECTION('center_axis',(0.,0.,-1.));
#45935=DIRECTION('ref_axis',(-1.,0.,0.));
#45936=DIRECTION('',(0.,0.,-1.));
#45937=DIRECTION('center_axis',(0.,0.,-1.));
#45938=DIRECTION('ref_axis',(-1.,0.,0.));
#45939=DIRECTION('',(0.,0.,-1.));
#45940=DIRECTION('',(0.,0.,-1.));
#45941=DIRECTION('center_axis',(0.,0.,-1.));
#45942=DIRECTION('ref_axis',(-1.,0.,0.));
#45943=DIRECTION('center_axis',(-1.,0.,0.));
#45944=DIRECTION('ref_axis',(0.,0.,1.));
#45945=DIRECTION('',(0.,0.,-1.));
#45946=DIRECTION('',(0.,-1.,0.));
#45947=DIRECTION('',(0.,1.,0.));
#45948=DIRECTION('center_axis',(0.,0.,-1.));
#45949=DIRECTION('ref_axis',(-1.,0.,0.));
#45950=DIRECTION('',(0.,0.,-1.));
#45951=DIRECTION('center_axis',(0.,0.,-1.));
#45952=DIRECTION('ref_axis',(-1.,0.,0.));
#45953=DIRECTION('center_axis',(0.,0.,-1.));
#45954=DIRECTION('ref_axis',(-1.,0.,0.));
#45955=DIRECTION('',(0.,0.,-1.));
#45956=DIRECTION('center_axis',(0.,1.,0.));
#45957=DIRECTION('ref_axis',(0.,0.,1.));
#45958=DIRECTION('',(1.,0.,0.));
#45959=DIRECTION('center_axis',(0.,0.,-1.));
#45960=DIRECTION('ref_axis',(-1.,0.,0.));
#45961=DIRECTION('',(0.,0.,-1.));
#45962=DIRECTION('center_axis',(0.,0.,-1.));
#45963=DIRECTION('ref_axis',(-1.,0.,0.));
#45964=DIRECTION('center_axis',(0.,0.,-1.));
#45965=DIRECTION('ref_axis',(-1.,0.,0.));
#45966=DIRECTION('',(0.,0.,-1.));
#45967=DIRECTION('center_axis',(-1.52617206349959E-16,-1.,0.));
#45968=DIRECTION('ref_axis',(1.,-1.52617206349959E-16,0.));
#45969=DIRECTION('',(-1.,1.52617206349959E-16,0.));
#45970=DIRECTION('center_axis',(0.563591301375832,-0.82605377852383,0.));
#45971=DIRECTION('ref_axis',(0.82605377852383,0.563591301375832,0.));
#45972=DIRECTION('',(0.,0.,-1.));
#45973=DIRECTION('',(-0.82605377852383,-0.563591301375832,0.));
#45974=DIRECTION('center_axis',(0.,0.,-1.));
#45975=DIRECTION('ref_axis',(1.,-3.21624529935327E-16,0.));
#45976=DIRECTION('',(0.,0.,-1.));
#45977=DIRECTION('center_axis',(0.,0.,-1.));
#45978=DIRECTION('ref_axis',(-1.,0.,0.));
#45979=DIRECTION('center_axis',(0.563591301375832,0.826053778523829,0.));
#45980=DIRECTION('ref_axis',(-0.82605377852383,0.563591301375832,0.));
#45981=DIRECTION('',(0.826053778523829,-0.563591301375832,0.));
#45982=DIRECTION('center_axis',(0.,0.,-1.));
#45983=DIRECTION('ref_axis',(-1.,0.,0.));
#45984=DIRECTION('center_axis',(0.563591301375832,-0.826053778523829,0.));
#45985=DIRECTION('ref_axis',(0.82605377852383,0.563591301375832,0.));
#45986=DIRECTION('',(-0.826053778523829,-0.563591301375832,0.));
#45987=DIRECTION('center_axis',(0.563591301375832,0.82605377852383,0.));
#45988=DIRECTION('ref_axis',(-0.82605377852383,0.563591301375832,0.));
#45989=DIRECTION('',(0.82605377852383,-0.563591301375832,0.));
#45990=DIRECTION('center_axis',(0.,0.,-1.));
#45991=DIRECTION('ref_axis',(-1.,0.,0.));
#45992=DIRECTION('center_axis',(0.,0.,-1.));
#45993=DIRECTION('ref_axis',(-1.,0.,0.));
#45994=DIRECTION('center_axis',(-1.,0.,0.));
#45995=DIRECTION('ref_axis',(0.,0.,1.));
#45996=DIRECTION('center_axis',(-6.82961998416064E-15,-1.,-6.82961998416066E-15));
#45997=DIRECTION('ref_axis',(-3.33169350914619E-30,6.82961998416066E-15,
-1.));
#45998=DIRECTION('center_axis',(0.,1.,0.));
#45999=DIRECTION('ref_axis',(0.,0.,1.));
#46000=DIRECTION('center_axis',(0.,-1.,-6.82961998416066E-15));
#46001=DIRECTION('ref_axis',(0.,6.82961998416066E-15,-1.));
#46002=DIRECTION('center_axis',(-1.,0.,0.));
#46003=DIRECTION('ref_axis',(0.,0.,1.));
#46004=DIRECTION('center_axis',(-1.,6.82961998416066E-15,0.));
#46005=DIRECTION('ref_axis',(-6.82961998416066E-15,-1.,0.));
#46006=DIRECTION('center_axis',(0.,0.,-1.));
#46007=DIRECTION('ref_axis',(-1.,0.,0.));
#46008=DIRECTION('center_axis',(-1.,6.82961998416066E-15,-6.82961998416066E-15));
#46009=DIRECTION('ref_axis',(-6.82961998416066E-15,1.33267740365848E-29,
1.));
#46010=DIRECTION('center_axis',(0.,0.,-1.));
#46011=DIRECTION('ref_axis',(-1.,0.,0.));
#46012=DIRECTION('center_axis',(0.,-1.,0.));
#46013=DIRECTION('ref_axis',(0.,0.,-1.));
#46014=DIRECTION('center_axis',(1.,-1.52617206349959E-16,0.));
#46015=DIRECTION('ref_axis',(1.52617206349959E-16,1.,0.));
#46016=DIRECTION('center_axis',(-1.,0.,-6.82961998416066E-15));
#46017=DIRECTION('ref_axis',(-6.82961998416066E-15,0.,1.));
#46018=DIRECTION('center_axis',(0.,-1.,0.));
#46019=DIRECTION('ref_axis',(0.,0.,-1.));
#46020=DIRECTION('center_axis',(-6.82961998416064E-15,-1.,0.));
#46021=DIRECTION('ref_axis',(1.,-6.82961998416064E-15,0.));
#46022=DIRECTION('center_axis',(0.,0.,-1.));
#46023=DIRECTION('ref_axis',(-1.,0.,0.));
#46024=DIRECTION('center_axis',(0.,0.,1.));
#46025=DIRECTION('ref_axis',(1.,0.,0.));
#46026=DIRECTION('',(0.,0.,1.));
#46027=DIRECTION('',(0.,0.,1.));
#46028=DIRECTION('center_axis',(0.,-1.,0.));
#46029=DIRECTION('ref_axis',(0.,0.,-1.));
#46030=DIRECTION('',(0.,0.,1.));
#46031=DIRECTION('center_axis',(0.,0.,1.));
#46032=DIRECTION('ref_axis',(1.,0.,0.));
#46033=DIRECTION('',(0.,0.,1.));
#46034=DIRECTION('center_axis',(1.,2.33197918015441E-16,0.));
#46035=DIRECTION('ref_axis',(-2.33197918015441E-16,1.,0.));
#46036=DIRECTION('',(0.,0.,1.));
#46037=DIRECTION('center_axis',(0.,0.,1.));
#46038=DIRECTION('ref_axis',(1.,0.,0.));
#46039=DIRECTION('',(0.,0.,1.));
#46040=DIRECTION('center_axis',(-0.707106781186552,0.707106781186543,0.));
#46041=DIRECTION('ref_axis',(-0.707106781186543,-0.707106781186552,0.));
#46042=DIRECTION('',(0.,0.,1.));
#46043=DIRECTION('center_axis',(0.,0.,1.));
#46044=DIRECTION('ref_axis',(1.,0.,0.));
#46045=DIRECTION('',(0.,0.,1.));
#46046=DIRECTION('center_axis',(3.20838317005448E-16,1.,0.));
#46047=DIRECTION('ref_axis',(-1.,3.20838317005448E-16,0.));
#46048=DIRECTION('',(0.,0.,1.));
#46049=DIRECTION('center_axis',(0.,0.,1.));
#46050=DIRECTION('ref_axis',(1.,0.,0.));
#46051=DIRECTION('',(0.,0.,1.));
#46052=DIRECTION('center_axis',(-0.707106781186551,-0.707106781186544,0.));
#46053=DIRECTION('ref_axis',(0.707106781186544,-0.707106781186551,0.));
#46054=DIRECTION('',(0.,0.,1.));
#46055=DIRECTION('center_axis',(0.,0.,1.));
#46056=DIRECTION('ref_axis',(1.,0.,0.));
#46057=DIRECTION('',(0.,0.,1.));
#46058=DIRECTION('center_axis',(-1.,-2.33197918015441E-16,0.));
#46059=DIRECTION('ref_axis',(2.33197918015441E-16,-1.,0.));
#46060=DIRECTION('center_axis',(0.,0.,1.));
#46061=DIRECTION('ref_axis',(1.,0.,0.));
#46062=DIRECTION('',(0.,0.,1.));
#46063=DIRECTION('',(0.,0.,1.));
#46064=DIRECTION('center_axis',(-0.707106781186551,-0.707106781186544,0.));
#46065=DIRECTION('ref_axis',(0.707106781186544,-0.707106781186551,0.));
#46066=DIRECTION('',(0.,0.,1.));
#46067=DIRECTION('center_axis',(0.,0.,1.));
#46068=DIRECTION('ref_axis',(1.,0.,0.));
#46069=DIRECTION('',(0.,0.,1.));
#46070=DIRECTION('center_axis',(-1.,0.,0.));
#46071=DIRECTION('ref_axis',(0.,0.,1.));
#46072=DIRECTION('',(0.,0.,1.));
#46073=DIRECTION('center_axis',(0.,0.,1.));
#46074=DIRECTION('ref_axis',(1.,0.,0.));
#46075=DIRECTION('',(0.,0.,1.));
#46076=DIRECTION('center_axis',(0.,-1.,0.));
#46077=DIRECTION('ref_axis',(0.,0.,-1.));
#46078=DIRECTION('',(0.,0.,1.));
#46079=DIRECTION('center_axis',(0.,0.,1.));
#46080=DIRECTION('ref_axis',(1.,0.,0.));
#46081=DIRECTION('',(0.,0.,1.));
#46082=DIRECTION('center_axis',(1.,0.,0.));
#46083=DIRECTION('ref_axis',(0.,0.,-1.));
#46084=DIRECTION('',(0.,0.,1.));
#46085=DIRECTION('center_axis',(0.,0.,1.));
#46086=DIRECTION('ref_axis',(1.,0.,0.));
#46087=DIRECTION('',(0.,0.,1.));
#46088=DIRECTION('center_axis',(-0.707106781186551,0.707106781186544,0.));
#46089=DIRECTION('ref_axis',(-0.707106781186544,-0.707106781186551,0.));
#46090=DIRECTION('',(0.,0.,1.));
#46091=DIRECTION('center_axis',(0.,0.,1.));
#46092=DIRECTION('ref_axis',(1.,0.,0.));
#46093=DIRECTION('',(0.,0.,1.));
#46094=DIRECTION('center_axis',(0.,1.,0.));
#46095=DIRECTION('ref_axis',(0.,0.,1.));
#46096=DIRECTION('center_axis',(-1.,0.,0.));
#46097=DIRECTION('ref_axis',(0.,0.,1.));
#46098=DIRECTION('',(0.,-1.,0.));
#46099=DIRECTION('center_axis',(-1.,-2.06958181338202E-16,0.));
#46100=DIRECTION('ref_axis',(2.06958181338202E-16,-1.,0.));
#46101=DIRECTION('',(2.06958181338202E-16,-1.,-9.33528028464659E-16));
#46102=DIRECTION('center_axis',(1.,-6.20874544014605E-16,0.));
#46103=DIRECTION('ref_axis',(6.20874544014605E-16,1.,0.));
#46104=DIRECTION('',(6.20874544014605E-16,1.,-2.80058408539397E-15));
#46105=DIRECTION('center_axis',(-0.976296007119933,0.,-0.216439613938103));
#46106=DIRECTION('ref_axis',(-0.216439613938103,0.,0.976296007119933));
#46107=DIRECTION('center_axis',(-0.976296007119933,0.,0.216439613938103));
#46108=DIRECTION('ref_axis',(0.216439613938103,0.,0.976296007119933));
#46109=DIRECTION('center_axis',(-0.976296007119933,0.,-0.216439613938104));
#46110=DIRECTION('ref_axis',(-0.216439613938104,0.,0.976296007119933));
#46111=DIRECTION('center_axis',(-0.976296007119933,0.,0.216439613938104));
#46112=DIRECTION('ref_axis',(0.216439613938104,0.,0.976296007119933));
#46113=DIRECTION('center_axis',(-0.94498615456937,0.,0.327110329510081));
#46114=DIRECTION('ref_axis',(0.327110329510081,0.,0.944986154569371));
#46115=DIRECTION('center_axis',(-0.94498615456937,0.,-0.327110329510081));
#46116=DIRECTION('ref_axis',(-0.327110329510081,0.,0.944986154569371));
#46117=DIRECTION('center_axis',(0.,0.,1.));
#46118=DIRECTION('ref_axis',(1.,0.,0.));
#46119=DIRECTION('',(1.,0.,0.));
#46120=DIRECTION('',(6.96899998383741E-17,1.,0.));
#46121=DIRECTION('',(-1.,0.,0.));
#46122=DIRECTION('',(1.39379999676748E-16,-1.,0.));
#46123=DIRECTION('',(-1.,-6.72614310123308E-16,0.));
#46124=DIRECTION('',(-2.06958181338202E-16,-1.,0.));
#46125=DIRECTION('',(1.,0.,0.));
#46126=DIRECTION('',(1.29348863336376E-16,-1.,0.));
#46127=DIRECTION('center_axis',(0.,-1.,0.));
#46128=DIRECTION('ref_axis',(0.,0.,-1.));
#46129=DIRECTION('',(0.,0.,1.));
#46130=DIRECTION('',(0.,0.,1.));
#46131=DIRECTION('center_axis',(1.,-6.96899998383741E-17,0.));
#46132=DIRECTION('ref_axis',(6.96899998383741E-17,1.,0.));
#46133=DIRECTION('',(0.,0.,1.));
#46134=DIRECTION('center_axis',(0.,1.,0.));
#46135=DIRECTION('ref_axis',(0.,0.,1.));
#46136=DIRECTION('',(0.,0.,1.));
#46137=DIRECTION('center_axis',(-1.,-1.39379999676748E-16,0.));
#46138=DIRECTION('ref_axis',(1.39379999676748E-16,-1.,0.));
#46139=DIRECTION('center_axis',(0.,0.707106781186548,-0.707106781186547));
#46140=DIRECTION('ref_axis',(0.,0.707106781186547,0.707106781186548));
#46141=DIRECTION('',(1.46341533446278E-16,0.707106781186547,0.707106781186548));
#46142=DIRECTION('',(1.,6.72614310123308E-16,6.7261431012331E-16));
#46143=DIRECTION('',(-9.14634584039234E-17,0.707106781186547,0.707106781186548));
#46144=DIRECTION('',(-1.,0.,0.));
#46145=DIRECTION('center_axis',(0.,0.,1.));
#46146=DIRECTION('ref_axis',(1.,0.,0.));
#46147=DIRECTION('',(-1.29348863336376E-16,1.,0.));
#46148=DIRECTION('',(-1.,0.,0.));
#46149=DIRECTION('',(2.06958181338202E-16,1.,0.));
#46150=DIRECTION('center_axis',(0.,0.707106781186547,0.707106781186548));
#46151=DIRECTION('ref_axis',(0.,-0.707106781186548,0.707106781186547));
#46152=DIRECTION('',(-1.46341533446278E-16,-0.707106781186548,0.707106781186547));
#46153=DIRECTION('',(9.14634584039236E-17,-0.707106781186548,0.707106781186547));
#46154=DIRECTION('',(1.,0.,0.));
#46155=DIRECTION('center_axis',(0.,1.,0.));
#46156=DIRECTION('ref_axis',(0.,0.,1.));
#46157=DIRECTION('',(0.,0.,1.));
#46158=DIRECTION('',(0.,0.,1.));
#46159=DIRECTION('center_axis',(1.,1.29348863336376E-16,0.));
#46160=DIRECTION('ref_axis',(-1.29348863336376E-16,1.,0.));
#46161=DIRECTION('',(0.,0.,1.));
#46162=DIRECTION('center_axis',(6.72614310123308E-16,-1.,0.));
#46163=DIRECTION('ref_axis',(1.,6.72614310123308E-16,0.));
#46164=DIRECTION('',(0.,0.,1.));
#46165=DIRECTION('center_axis',(1.,-2.06958181338202E-16,0.));
#46166=DIRECTION('ref_axis',(2.06958181338202E-16,1.,0.));
#46167=DIRECTION('center_axis',(0.,-1.,0.));
#46168=DIRECTION('ref_axis',(0.,0.,-1.));
#46169=DIRECTION('',(0.,0.,1.));
#46170=DIRECTION('',(1.,0.,0.));
#46171=DIRECTION('',(0.,0.,1.));
#46172=DIRECTION('center_axis',(1.,-2.78759999353496E-16,0.));
#46173=DIRECTION('ref_axis',(2.78759999353496E-16,1.,0.));
#46174=DIRECTION('',(0.,0.,1.));
#46175=DIRECTION('',(2.78759999353496E-16,1.,0.));
#46176=DIRECTION('center_axis',(-6.44303772090628E-16,1.,0.));
#46177=DIRECTION('ref_axis',(-1.,-6.44303772090628E-16,0.));
#46178=DIRECTION('',(0.,0.,1.));
#46179=DIRECTION('',(-1.,-6.44303772090628E-16,0.));
#46180=DIRECTION('center_axis',(-1.,2.78759999353496E-16,0.));
#46181=DIRECTION('ref_axis',(-2.78759999353496E-16,-1.,0.));
#46182=DIRECTION('',(-2.78759999353496E-16,-1.,0.));
#46183=DIRECTION('center_axis',(0.,0.,-1.));
#46184=DIRECTION('ref_axis',(-1.,0.,0.));
#46185=DIRECTION('',(0.,-1.,0.));
#46186=DIRECTION('',(-1.,0.,0.));
#46187=DIRECTION('',(0.,-1.,0.));
#46188=DIRECTION('',(1.,0.,0.));
#46189=DIRECTION('center_axis',(0.,0.,1.));
#46190=DIRECTION('ref_axis',(1.,0.,0.));
#46191=DIRECTION('',(0.,-1.,0.));
#46192=DIRECTION('',(-1.,0.,0.));
#46193=DIRECTION('',(0.,-1.,0.));
#46194=DIRECTION('',(-1.,0.,0.));
#46195=DIRECTION('center_axis',(0.,0.707106781186547,-0.707106781186548));
#46196=DIRECTION('ref_axis',(0.,0.707106781186548,0.707106781186547));
#46197=DIRECTION('',(0.,0.707106781186548,0.707106781186547));
#46198=DIRECTION('',(0.,-0.707106781186548,-0.707106781186547));
#46199=DIRECTION('',(-1.,0.,0.));
#46200=DIRECTION('center_axis',(0.,0.707106781186548,0.707106781186547));
#46201=DIRECTION('ref_axis',(0.,-0.707106781186547,0.707106781186548));
#46202=DIRECTION('',(-1.,0.,0.));
#46203=DIRECTION('',(0.,0.707106781186547,-0.707106781186548));
#46204=DIRECTION('',(0.,-0.707106781186547,0.707106781186548));
#46205=DIRECTION('center_axis',(0.,-1.,0.));
#46206=DIRECTION('ref_axis',(0.,0.,-1.));
#46207=DIRECTION('',(0.,0.,1.));
#46208=DIRECTION('',(0.,0.,1.));
#46209=DIRECTION('center_axis',(0.,1.,0.));
#46210=DIRECTION('ref_axis',(0.,0.,1.));
#46211=DIRECTION('',(0.,0.,1.));
#46212=DIRECTION('',(0.,0.,1.));
#46213=DIRECTION('center_axis',(-1.,0.,0.));
#46214=DIRECTION('ref_axis',(0.,0.,1.));
#46215=DIRECTION('center_axis',(-1.,0.,0.));
#46216=DIRECTION('ref_axis',(0.,0.,1.));
#46217=DIRECTION('center_axis',(0.,0.,1.));
#46218=DIRECTION('ref_axis',(1.,0.,0.));
#46219=DIRECTION('',(-1.39379999676748E-16,1.,0.));
#46220=DIRECTION('',(-1.,0.,0.));
#46221=DIRECTION('',(5.57519998706993E-16,-1.,0.));
#46222=DIRECTION('',(1.,6.44303772090628E-16,0.));
#46223=DIRECTION('',(0.,-1.,0.));
#46224=DIRECTION('',(-1.,0.,0.));
#46225=DIRECTION('',(0.,-1.,0.));
#46226=DIRECTION('',(1.,0.,0.));
#46227=DIRECTION('center_axis',(1.,1.39379999676748E-16,0.));
#46228=DIRECTION('ref_axis',(-1.39379999676748E-16,1.,0.));
#46229=DIRECTION('',(0.,0.,1.));
#46230=DIRECTION('',(0.,0.,1.));
#46231=DIRECTION('center_axis',(0.,1.,0.));
#46232=DIRECTION('ref_axis',(0.,0.,1.));
#46233=DIRECTION('',(0.,0.,1.));
#46234=DIRECTION('center_axis',(-1.,-5.57519998706993E-16,0.));
#46235=DIRECTION('ref_axis',(5.57519998706993E-16,-1.,0.));
#46236=DIRECTION('',(0.,0.,1.));
#46237=DIRECTION('center_axis',(6.44303772090628E-16,-1.,0.));
#46238=DIRECTION('ref_axis',(1.,6.44303772090628E-16,0.));
#46239=DIRECTION('center_axis',(0.,0.,-1.));
#46240=DIRECTION('ref_axis',(-1.,0.,0.));
#46241=DIRECTION('',(1.,0.,0.));
#46242=DIRECTION('',(0.,1.,0.));
#46243=DIRECTION('',(1.,0.,0.));
#46244=DIRECTION('',(0.,1.,0.));
#46245=DIRECTION('center_axis',(0.,0.707106781186547,-0.707106781186548));
#46246=DIRECTION('ref_axis',(0.,0.707106781186548,0.707106781186547));
#46247=DIRECTION('',(1.,0.,0.));
#46248=DIRECTION('',(0.,0.707106781186548,0.707106781186547));
#46249=DIRECTION('',(0.,0.707106781186548,0.707106781186547));
#46250=DIRECTION('center_axis',(0.,0.707106781186548,0.707106781186547));
#46251=DIRECTION('ref_axis',(0.,-0.707106781186547,0.707106781186548));
#46252=DIRECTION('',(0.,-0.707106781186547,0.707106781186548));
#46253=DIRECTION('',(1.,0.,0.));
#46254=DIRECTION('',(0.,-0.707106781186547,0.707106781186548));
#46255=DIRECTION('center_axis',(0.,1.,0.));
#46256=DIRECTION('ref_axis',(0.,0.,1.));
#46257=DIRECTION('',(0.,0.,1.));
#46258=DIRECTION('',(0.,0.,1.));
#46259=DIRECTION('center_axis',(0.,-1.,0.));
#46260=DIRECTION('ref_axis',(0.,0.,-1.));
#46261=DIRECTION('',(0.,0.,1.));
#46262=DIRECTION('',(0.,0.,1.));
#46263=DIRECTION('center_axis',(1.,0.,0.));
#46264=DIRECTION('ref_axis',(0.,0.,-1.));
#46265=DIRECTION('center_axis',(1.,0.,0.));
#46266=DIRECTION('ref_axis',(0.,0.,-1.));
#57363=CARTESIAN_POINT('',(0.,0.,0.));
#57364=CARTESIAN_POINT('Origin',(-17.78,1.7549973081547,-14.4736733188239));
#57365=CARTESIAN_POINT('',(-5.01908361227606,1.7549973081547,-13.6735733188239));
#57366=CARTESIAN_POINT('Origin',(-5.01908361227606,1.7549973081547,-14.4736733188239));
#57367=CARTESIAN_POINT('',(-4.24429638772394,1.7549973081547,-13.6735733188239));
#57368=CARTESIAN_POINT('',(-17.78,1.7549973081547,-13.6735733188239));
#57369=CARTESIAN_POINT('Origin',(-4.24429638772394,1.7549973081547,-14.4736733188239));
#57370=CARTESIAN_POINT('Origin',(-17.78,1.7549973081547,-14.4736733188239));
#57371=CARTESIAN_POINT('',(4.24429638772393,1.7549973081547,-13.6735733188239));
#57372=CARTESIAN_POINT('Origin',(4.24429638772394,1.7549973081547,-14.4736733188239));
#57373=CARTESIAN_POINT('',(5.01908361227606,1.7549973081547,-13.6735733188239));
#57374=CARTESIAN_POINT('',(-17.78,1.7549973081547,-13.6735733188239));
#57375=CARTESIAN_POINT('Origin',(5.01908361227606,1.7549973081547,-14.4736733188239));
#57376=CARTESIAN_POINT('Origin',(-17.78,-1.6232026918453,-14.4736733188239));
#57377=CARTESIAN_POINT('',(-0.451338313394325,-1.6232026918453,-13.6735733188239));
#57378=CARTESIAN_POINT('Origin',(-0.451338313394324,-1.6232026918453,-14.4736733188239));
#57379=CARTESIAN_POINT('',(0.451338313394325,-1.6232026918453,-13.6735733188239));
#57380=CARTESIAN_POINT('',(-17.78,-1.6232026918453,-13.6735733188239));
#57381=CARTESIAN_POINT('Origin',(0.451338313394325,-1.6232026918453,-14.4736733188239));
#57382=CARTESIAN_POINT('Origin',(-14.224,0.0658973081546998,1.33274668117609));
#57383=CARTESIAN_POINT('',(-13.02385,0.0658973081546999,0.443746681176088));
#57384=CARTESIAN_POINT('',(-15.42415,0.0658973081546997,0.443746681176088));
#57385=CARTESIAN_POINT('Origin',(-14.224,0.0658973081546998,0.443746681176088));
#57386=CARTESIAN_POINT('Origin',(-14.224,0.0658973081546998,0.443746681176088));
#57387=CARTESIAN_POINT('',(-16.1969459099186,0.0658973081546996,1.33274668117609));
#57388=CARTESIAN_POINT('',(-16.1969459099186,0.0658973081546996,1.33274668117609));
#57389=CARTESIAN_POINT('Origin',(-14.224,0.0658973081546998,1.33274668117609));
#57390=CARTESIAN_POINT('Origin',(14.224,0.0658973081546998,1.33274668117609));
#57391=CARTESIAN_POINT('',(15.42415,0.0658973081546999,0.443746681176088));
#57392=CARTESIAN_POINT('',(13.02385,0.0658973081546997,0.443746681176088));
#57393=CARTESIAN_POINT('Origin',(14.224,0.0658973081546998,0.443746681176088));
#57394=CARTESIAN_POINT('Origin',(14.224,0.0658973081546998,0.443746681176088));
#57395=CARTESIAN_POINT('',(12.2510540900814,0.0658973081546996,1.33274668117609));
#57396=CARTESIAN_POINT('',(12.2510540900814,0.0658973081546996,1.33274668117609));
#57397=CARTESIAN_POINT('Origin',(14.224,0.0658973081546998,1.33274668117609));
#57398=CARTESIAN_POINT('Origin',(-14.224,0.0658973081546998,1.33274668117609));
#57399=CARTESIAN_POINT('',(-13.02385,0.0658973081546997,-0.871973318823906));
#57400=CARTESIAN_POINT('',(-13.02385,0.0658973081546997,1.33274668117609));
#57401=CARTESIAN_POINT('Origin',(-14.224,0.0658973081546998,-0.871973318823906));
#57402=CARTESIAN_POINT('Origin',(-14.224,0.0658973081546998,1.33274668117609));
#57403=CARTESIAN_POINT('',(-16.2281306676925,3.00334454458544,1.33274668117609));
#57404=CARTESIAN_POINT('',(-16.2281306676925,-2.87154992827604,1.33274668117609));
#57405=CARTESIAN_POINT('Origin',(-14.224,0.0658973081546998,1.33274668117609));
#57406=CARTESIAN_POINT('',(-16.2281306676925,3.00334454458544,-0.871973318823906));
#57407=CARTESIAN_POINT('',(-16.2281306676925,3.00334454458544,1.33274668117609));
#57408=CARTESIAN_POINT('',(-16.2281306676925,-2.87154992827604,-0.871973318823906));
#57409=CARTESIAN_POINT('Origin',(-14.224,0.0658973081546998,-0.871973318823906));
#57410=CARTESIAN_POINT('',(-16.2281306676925,-2.87154992827604,1.33274668117609));
#57411=CARTESIAN_POINT('Origin',(14.224,0.0658973081546998,1.33274668117609));
#57412=CARTESIAN_POINT('',(15.42415,0.0658973081546997,-0.871973318823906));
#57413=CARTESIAN_POINT('',(15.42415,0.0658973081546997,1.33274668117609));
#57414=CARTESIAN_POINT('Origin',(14.224,0.0658973081546998,-0.871973318823906));
#57415=CARTESIAN_POINT('Origin',(-6.6675,4.1108473081547,-10.0286733188239));
#57416=CARTESIAN_POINT('',(-9.3345,4.11084730815468,-10.0286733188239));
#57417=CARTESIAN_POINT('',(-6.66749999999998,6.7778473081547,-10.0286733188239));
#57418=CARTESIAN_POINT('Origin',(-6.6675,4.1108473081547,-10.0286733188239));
#57419=CARTESIAN_POINT('',(6.66749999999998,6.7778473081547,-10.0286733188239));
#57420=CARTESIAN_POINT('',(-6.66749999999998,6.7778473081547,-10.0286733188239));
#57421=CARTESIAN_POINT('',(9.3345,4.11084730815468,-10.0286733188239));
#57422=CARTESIAN_POINT('Origin',(6.6675,4.1108473081547,-10.0286733188239));
#57423=CARTESIAN_POINT('',(9.3345,-1.09634512099626,-10.0286733188239));
#57424=CARTESIAN_POINT('',(9.3345,-1.09634512099627,-10.0286733188239));
#57425=CARTESIAN_POINT('',(8.55335378542453,-2.98219890642078,-10.0286733188239));
#57426=CARTESIAN_POINT('Origin',(6.6675,-1.09634512099626,-10.0286733188239));
#57427=CARTESIAN_POINT('',(5.67064621457553,-5.86490647726981,-10.0286733188239));
#57428=CARTESIAN_POINT('',(8.55335378542453,-2.98219890642078,-10.0286733188239));
#57429=CARTESIAN_POINT('',(3.784792429151,-6.6460526918453,-10.0286733188239));
#57430=CARTESIAN_POINT('Origin',(3.78479242915099,-3.9790526918453,-10.0286733188239));
#57431=CARTESIAN_POINT('',(-3.78479242915098,-6.6460526918453,-10.0286733188239));
#57432=CARTESIAN_POINT('',(3.784792429151,-6.6460526918453,-10.0286733188239));
#57433=CARTESIAN_POINT('',(-5.67064621457553,-5.8649064772698,-10.0286733188239));
#57434=CARTESIAN_POINT('Origin',(-3.78479242915099,-3.9790526918453,-10.0286733188239));
#57435=CARTESIAN_POINT('',(-8.55335378542452,-2.98219890642078,-10.0286733188239));
#57436=CARTESIAN_POINT('',(-8.55335378542452,-2.98219890642078,-10.0286733188239));
#57437=CARTESIAN_POINT('',(-9.3345,-1.09634512099625,-10.0286733188239));
#57438=CARTESIAN_POINT('Origin',(-6.6675,-1.09634512099626,-10.0286733188239));
#57439=CARTESIAN_POINT('',(-9.3345,4.11084730815468,-10.0286733188239));
#57440=CARTESIAN_POINT('',(1.41351,-3.8012526918453,-10.0286733188239));
#57441=CARTESIAN_POINT('',(1.41351,0.554847308154699,-10.0286733188239));
#57442=CARTESIAN_POINT('',(1.41351,-3.8012526918453,-10.0286733188239));
#57443=CARTESIAN_POINT('',(-1.41351,0.554847308154699,-10.0286733188239));
#57444=CARTESIAN_POINT('',(-1.41351,0.554847308154699,-10.0286733188239));
#57445=CARTESIAN_POINT('',(-1.41351,-3.8012526918453,-10.0286733188239));
#57446=CARTESIAN_POINT('',(-1.41351,0.554847308154699,-10.0286733188239));
#57447=CARTESIAN_POINT('',(1.41351,-3.8012526918453,-10.0286733188239));
#57448=CARTESIAN_POINT('',(-3.21818,-0.4230526918453,-10.0286733188239));
#57449=CARTESIAN_POINT('',(-3.21818,3.9330473081547,-10.0286733188239));
#57450=CARTESIAN_POINT('',(-3.21818,-0.4230526918453,-10.0286733188239));
#57451=CARTESIAN_POINT('',(-6.0452,3.9330473081547,-10.0286733188239));
#57452=CARTESIAN_POINT('',(-6.0452,3.9330473081547,-10.0286733188239));
#57453=CARTESIAN_POINT('',(-6.0452,-0.4230526918453,-10.0286733188239));
#57454=CARTESIAN_POINT('',(-6.0452,3.9330473081547,-10.0286733188239));
#57455=CARTESIAN_POINT('',(-3.21818,-0.4230526918453,-10.0286733188239));
#57456=CARTESIAN_POINT('',(3.21818,-0.4230526918453,-10.0286733188239));
#57457=CARTESIAN_POINT('',(6.0452,-0.4230526918453,-10.0286733188239));
#57458=CARTESIAN_POINT('',(3.21818,-0.4230526918453,-10.0286733188239));
#57459=CARTESIAN_POINT('',(6.0452,3.9330473081547,-10.0286733188239));
#57460=CARTESIAN_POINT('',(6.0452,3.9330473081547,-10.0286733188239));
#57461=CARTESIAN_POINT('',(3.21818,3.9330473081547,-10.0286733188239));
#57462=CARTESIAN_POINT('',(6.0452,3.9330473081547,-10.0286733188239));
#57463=CARTESIAN_POINT('',(3.21818,-0.4230526918453,-10.0286733188239));
#57464=CARTESIAN_POINT('Origin',(-0.70231,-0.156352691845301,0.194826681176092));
#57465=CARTESIAN_POINT('',(-0.70231,-0.156352691845301,2.11901678258961));
#57466=CARTESIAN_POINT('',(-0.70231,-3.0900526918453,2.11901678258961));
#57467=CARTESIAN_POINT('',(-0.70231,-0.1563526918453,2.11901678258961));
#57468=CARTESIAN_POINT('',(-0.70231,-0.156352691845301,-8.4284733188239));
#57469=CARTESIAN_POINT('',(-0.70231,-0.156352691845301,0.194826681176092));
#57470=CARTESIAN_POINT('',(-0.70231,-3.0900526918453,-8.4284733188239));
#57471=CARTESIAN_POINT('',(-0.702309999999999,-3.7123526918453,-8.42847331882391));
#57472=CARTESIAN_POINT('',(-0.70231,-3.0900526918453,0.194826681176092));
#57473=CARTESIAN_POINT('Origin',(0.70231,-3.0900526918453,0.194826681176092));
#57474=CARTESIAN_POINT('',(0.451338313394325,-3.0900526918453,2.84404668117609));
#57475=CARTESIAN_POINT('',(0.70231,-3.0900526918453,2.11901678258961));
#57476=CARTESIAN_POINT('',(0.2667,-3.0900526918453,3.37744668117609));
#57477=CARTESIAN_POINT('',(-0.451338313394325,-3.0900526918453,2.84404668117609));
#57478=CARTESIAN_POINT('',(-0.70231,-3.0900526918453,2.84404668117609));
#57479=CARTESIAN_POINT('',(-0.2667,-3.0900526918453,3.37744668117609));
#57480=CARTESIAN_POINT('',(0.70231,-3.0900526918453,-8.4284733188239));
#57481=CARTESIAN_POINT('',(-4.15302828610066,-3.0900526918453,-8.42847331882391));
#57482=CARTESIAN_POINT('',(0.70231,-3.0900526918453,0.194826681176092));
#57483=CARTESIAN_POINT('Origin',(-0.70231,-0.156352691845301,0.194826681176092));
#57484=CARTESIAN_POINT('',(0.451338313394325,-0.156352691845301,2.84404668117609));
#57485=CARTESIAN_POINT('',(0.70231,-0.156352691845301,2.11901678258961));
#57486=CARTESIAN_POINT('',(0.2667,-0.156352691845301,3.37744668117609));
#57487=CARTESIAN_POINT('',(0.70231,-0.156352691845301,-8.42847331882391));
#57488=CARTESIAN_POINT('',(0.70231,-0.156352691845301,0.194826681176092));
#57489=CARTESIAN_POINT('',(-4.15302828610066,-0.156352691845301,-8.42847331882391));
#57490=CARTESIAN_POINT('',(-0.451338313394325,-0.156352691845301,2.84404668117609));
#57491=CARTESIAN_POINT('',(-0.2667,-0.156352691845301,3.37744668117609));
#57492=CARTESIAN_POINT('',(0.70231,-0.156352691845301,2.84404668117609));
#57493=CARTESIAN_POINT('Origin',(7.95655,-4.2101926918453,2.84404668117609));
#57494=CARTESIAN_POINT('',(0.451338313394325,-4.2101926918453,2.84404668117609));
#57495=CARTESIAN_POINT('',(-0.451338313394325,-4.2101926918453,2.84404668117609));
#57496=CARTESIAN_POINT('Origin',(5.334,3.2218473081547,0.194826681176092));
#57497=CARTESIAN_POINT('',(4.24429638772394,3.2218473081547,0.194826681176092));
#57498=CARTESIAN_POINT('',(3.92938,3.2218473081547,-1.22566934687279));
#57499=CARTESIAN_POINT('',(4.29534475917809,3.2218473081547,0.425091004392428));
#57500=CARTESIAN_POINT('',(5.01908361227606,3.2218473081547,0.194826681176092));
#57501=CARTESIAN_POINT('',(5.334,3.2218473081547,0.194826681176092));
#57502=CARTESIAN_POINT('',(5.334,3.2218473081547,-1.2256693468728));
#57503=CARTESIAN_POINT('',(5.0338362189082,3.2218473081547,0.128281972989317));
#57504=CARTESIAN_POINT('',(5.334,3.2218473081547,-8.42847331882391));
#57505=CARTESIAN_POINT('',(5.334,3.2218473081547,0.194826681176092));
#57506=CARTESIAN_POINT('',(3.92938,3.2218473081547,-8.42847331882391));
#57507=CARTESIAN_POINT('',(-4.15302828610066,3.2218473081547,-8.42847331882391));
#57508=CARTESIAN_POINT('',(3.92938,3.2218473081547,0.194826681176092));
#57509=CARTESIAN_POINT('Origin',(3.92938,0.2881473081547,0.194826681176092));
#57510=CARTESIAN_POINT('',(3.92938,0.2881473081547,-1.2256693468728));
#57511=CARTESIAN_POINT('',(3.92938,0.2881473081547,-8.42847331882391));
#57512=CARTESIAN_POINT('',(3.92938,0.2881473081547,0.194826681176092));
#57513=CARTESIAN_POINT('',(3.92938,0.288147308154702,-1.2256693468728));
#57514=CARTESIAN_POINT('',(3.92938,-3.7123526918453,-8.42847331882391));
#57515=CARTESIAN_POINT('Origin',(3.92938,0.2881473081547,0.194826681176092));
#57516=CARTESIAN_POINT('',(4.24429638772394,0.2881473081547,0.194826681176092));
#57517=CARTESIAN_POINT('',(4.36283493912025,0.2881473081547,0.729519532971222));
#57518=CARTESIAN_POINT('',(5.334,0.2881473081547,-8.4284733188239));
#57519=CARTESIAN_POINT('',(-4.15302828610066,0.2881473081547,-8.42847331882391));
#57520=CARTESIAN_POINT('',(5.334,0.2881473081547,-1.22566934687279));
#57521=CARTESIAN_POINT('',(5.334,0.2881473081547,0.194826681176092));
#57522=CARTESIAN_POINT('',(5.01908361227606,0.2881473081547,0.194826681176092));
#57523=CARTESIAN_POINT('',(4.90054506087975,0.2881473081547,0.729519532971222));
#57524=CARTESIAN_POINT('',(3.92938,0.2881473081547,0.194826681176092));
#57525=CARTESIAN_POINT('Origin',(5.334,0.2881473081547,0.194826681176092));
#57526=CARTESIAN_POINT('',(4.24429638772394,0.2881473081547,0.194826681176092));
#57527=CARTESIAN_POINT('',(5.01908361227606,0.2881473081547,0.194826681176092));
#57528=CARTESIAN_POINT('Origin',(-5.334,3.2218473081547,0.194826681176092));
#57529=CARTESIAN_POINT('',(-5.334,3.2218473081547,-1.2256693468728));
#57530=CARTESIAN_POINT('',(-5.334,0.2881473081547,-1.22566934687279));
#57531=CARTESIAN_POINT('',(-5.334,3.2218473081547,-1.2256693468728));
#57532=CARTESIAN_POINT('',(-5.334,3.2218473081547,-8.4284733188239));
#57533=CARTESIAN_POINT('',(-5.334,3.2218473081547,0.194826681176092));
#57534=CARTESIAN_POINT('',(-5.334,0.2881473081547,-8.4284733188239));
#57535=CARTESIAN_POINT('',(-5.334,-3.7123526918453,-8.42847331882391));
#57536=CARTESIAN_POINT('',(-5.334,0.2881473081547,0.194826681176092));
#57537=CARTESIAN_POINT('Origin',(-3.92938,0.2881473081547,0.194826681176092));
#57538=CARTESIAN_POINT('',(-4.24429638772394,0.2881473081547,0.194826681176092));
#57539=CARTESIAN_POINT('',(-5.01908361227606,0.2881473081547,0.194826681176092));
#57540=CARTESIAN_POINT('',(-3.92938,0.2881473081547,0.194826681176092));
#57541=CARTESIAN_POINT('',(-4.90054506087975,0.2881473081547,0.729519532971223));
#57542=CARTESIAN_POINT('',(-3.92938,0.2881473081547,-8.4284733188239));
#57543=CARTESIAN_POINT('',(-4.15302828610066,0.2881473081547,-8.42847331882391));
#57544=CARTESIAN_POINT('',(-3.92938,0.2881473081547,-1.2256693468728));
#57545=CARTESIAN_POINT('',(-3.92938,0.2881473081547,0.194826681176092));
#57546=CARTESIAN_POINT('',(-4.36283493912025,0.2881473081547,0.729519532971223));
#57547=CARTESIAN_POINT('Origin',(-5.334,3.2218473081547,0.194826681176092));
#57548=CARTESIAN_POINT('',(-5.01908361227606,3.2218473081547,0.194826681176092));
#57549=CARTESIAN_POINT('',(-5.0338362189082,3.2218473081547,0.128281972989317));
#57550=CARTESIAN_POINT('',(-4.24429638772394,3.2218473081547,0.194826681176092));
#57551=CARTESIAN_POINT('',(-5.334,3.2218473081547,0.194826681176092));
#57552=CARTESIAN_POINT('',(-3.92938,3.2218473081547,-1.2256693468728));
#57553=CARTESIAN_POINT('',(-4.29534475917809,3.2218473081547,0.425091004392428));
#57554=CARTESIAN_POINT('',(-3.92938,3.2218473081547,-8.42847331882391));
#57555=CARTESIAN_POINT('',(-3.92938,3.2218473081547,0.194826681176092));
#57556=CARTESIAN_POINT('',(-4.15302828610066,3.2218473081547,-8.42847331882391));
#57557=CARTESIAN_POINT('Origin',(-5.334,0.2881473081547,0.194826681176092));
#57558=CARTESIAN_POINT('',(-5.01908361227606,0.2881473081547,0.194826681176092));
#57559=CARTESIAN_POINT('',(-4.24429638772394,0.2881473081547,0.194826681176092));
#57560=CARTESIAN_POINT('Origin',(-4.15302828610066,-3.7123526918453,-8.42847331882391));
#57561=CARTESIAN_POINT('',(-4.15302828610065,-5.4903526918453,-8.42847331882391));
#57562=CARTESIAN_POINT('',(-5.41026414305035,-4.96958854879497,-8.42847331882391));
#57563=CARTESIAN_POINT('Origin',(-4.15302828610066,-3.7123526918453,-8.42847331882391));
#57564=CARTESIAN_POINT('',(4.15302828610066,-5.4903526918453,-8.42847331882391));
#57565=CARTESIAN_POINT('',(4.15302828610066,-5.4903526918453,-8.42847331882391));
#57566=CARTESIAN_POINT('',(5.41026414305036,-4.96958854879497,-8.42847331882391));
#57567=CARTESIAN_POINT('Origin',(4.15302828610066,-3.7123526918453,-8.42847331882391));
#57568=CARTESIAN_POINT('',(7.92473585694968,-2.45511683489562,-8.42847331882391));
#57569=CARTESIAN_POINT('',(7.92473585694968,-2.45511683489562,-8.42847331882391));
#57570=CARTESIAN_POINT('',(8.4455,-1.19788097794593,-8.42847331882391));
#57571=CARTESIAN_POINT('Origin',(6.6675,-1.19788097794594,-8.42847331882391));
#57572=CARTESIAN_POINT('',(8.4455,3.84414730815469,-8.42847331882391));
#57573=CARTESIAN_POINT('',(8.4455,-1.19788097794593,-8.42847331882391));
#57574=CARTESIAN_POINT('',(6.66749999999999,5.6221473081547,-8.42847331882391));
#57575=CARTESIAN_POINT('Origin',(6.6675,3.8441473081547,-8.42847331882391));
#57576=CARTESIAN_POINT('',(-6.66749999999999,5.6221473081547,-8.42847331882391));
#57577=CARTESIAN_POINT('',(-6.66749999999999,5.6221473081547,-8.42847331882391));
#57578=CARTESIAN_POINT('',(-8.4455,3.84414730815469,-8.42847331882391));
#57579=CARTESIAN_POINT('Origin',(-6.6675,3.8441473081547,-8.42847331882391));
#57580=CARTESIAN_POINT('',(-8.4455,-1.19788097794593,-8.42847331882391));
#57581=CARTESIAN_POINT('',(-8.4455,3.84414730815469,-8.42847331882391));
#57582=CARTESIAN_POINT('',(-7.92473585694968,-2.45511683489562,-8.42847331882391));
#57583=CARTESIAN_POINT('Origin',(-6.6675,-1.19788097794594,-8.42847331882391));
#57584=CARTESIAN_POINT('',(-7.92473585694968,-2.45511683489562,-8.42847331882391));
#57585=CARTESIAN_POINT('',(-3.92938,-3.7123526918453,-8.42847331882391));
#57586=CARTESIAN_POINT('',(5.334,-3.71235269184531,-8.42847331882391));
#57587=CARTESIAN_POINT('',(0.70231,-3.7123526918453,-8.42847331882391));
#57588=CARTESIAN_POINT('Origin',(7.95655,-4.2101926918453,3.37744668117609));
#57589=CARTESIAN_POINT('',(-11.15695,4.34198730815467,3.37744668117609));
#57590=CARTESIAN_POINT('',(-11.15695,-4.21019269184528,3.37744668117609));
#57591=CARTESIAN_POINT('',(-11.15695,-4.2101926918453,3.37744668117609));
#57592=CARTESIAN_POINT('',(-7.95654999999997,-7.4105926918453,3.37744668117609));
#57593=CARTESIAN_POINT('Origin',(-7.95655,-4.2101926918453,3.37744668117609));
#57594=CARTESIAN_POINT('',(7.95654999999997,-7.4105926918453,3.37744668117609));
#57595=CARTESIAN_POINT('',(7.95654999999997,-7.4105926918453,3.37744668117609));
#57596=CARTESIAN_POINT('',(11.15695,-4.21019269184528,3.37744668117609));
#57597=CARTESIAN_POINT('Origin',(7.95655,-4.2101926918453,3.37744668117609));
#57598=CARTESIAN_POINT('',(11.15695,4.34198730815467,3.37744668117609));
#57599=CARTESIAN_POINT('',(11.15695,-4.2101926918453,3.37744668117609));
#57600=CARTESIAN_POINT('',(7.95654999999997,7.5423873081547,3.37744668117609));
#57601=CARTESIAN_POINT('Origin',(7.95655,4.3419873081547,3.37744668117609));
#57602=CARTESIAN_POINT('',(-7.95654999999997,7.5423873081547,3.37744668117609));
#57603=CARTESIAN_POINT('',(-7.95654999999997,7.5423873081547,3.37744668117609));
#57604=CARTESIAN_POINT('Origin',(-7.95655,4.3419873081547,3.37744668117609));
#57605=CARTESIAN_POINT('',(-4.15302828610065,-5.4903526918453,3.37744668117609));
#57606=CARTESIAN_POINT('',(-5.41026414305035,-4.96958854879497,3.37744668117609));
#57607=CARTESIAN_POINT('Origin',(-4.15302828610066,-3.7123526918453,3.37744668117609));
#57608=CARTESIAN_POINT('',(-7.92473585694968,-2.45511683489562,3.37744668117609));
#57609=CARTESIAN_POINT('',(-7.92473585694968,-2.45511683489562,3.37744668117609));
#57610=CARTESIAN_POINT('',(-8.4455,-1.19788097794593,3.37744668117609));
#57611=CARTESIAN_POINT('Origin',(-6.6675,-1.19788097794594,3.37744668117609));
#57612=CARTESIAN_POINT('',(-8.4455,3.84414730815469,3.37744668117609));
#57613=CARTESIAN_POINT('',(-8.4455,3.84414730815469,3.37744668117609));
#57614=CARTESIAN_POINT('',(-6.66749999999999,5.6221473081547,3.37744668117609));
#57615=CARTESIAN_POINT('Origin',(-6.6675,3.8441473081547,3.37744668117609));
#57616=CARTESIAN_POINT('',(6.66749999999999,5.6221473081547,3.37744668117609));
#57617=CARTESIAN_POINT('',(-6.66749999999999,5.6221473081547,3.37744668117609));
#57618=CARTESIAN_POINT('',(8.4455,3.84414730815469,3.37744668117609));
#57619=CARTESIAN_POINT('Origin',(6.6675,3.8441473081547,3.37744668117609));
#57620=CARTESIAN_POINT('',(8.4455,-1.19788097794593,3.37744668117609));
#57621=CARTESIAN_POINT('',(8.4455,-1.19788097794593,3.37744668117609));
#57622=CARTESIAN_POINT('',(7.92473585694968,-2.45511683489562,3.37744668117609));
#57623=CARTESIAN_POINT('Origin',(6.6675,-1.19788097794594,3.37744668117609));
#57624=CARTESIAN_POINT('',(5.41026414305036,-4.96958854879497,3.37744668117609));
#57625=CARTESIAN_POINT('',(7.92473585694968,-2.45511683489562,3.37744668117609));
#57626=CARTESIAN_POINT('',(4.15302828610066,-5.4903526918453,3.37744668117609));
#57627=CARTESIAN_POINT('Origin',(4.15302828610066,-3.7123526918453,3.37744668117609));
#57628=CARTESIAN_POINT('',(4.15302828610066,-5.4903526918453,3.37744668117609));
#57629=CARTESIAN_POINT('Origin',(7.95655,-4.2101926918453,-0.871973318823906));
#57630=CARTESIAN_POINT('',(-9.96068066769246,7.27943454458544,-0.871973318823906));
#57631=CARTESIAN_POINT('',(-9.96068066769246,7.27943454458544,-0.871973318823906));
#57632=CARTESIAN_POINT('',(-7.95654999999997,7.8979873081547,-0.871973318823906));
#57633=CARTESIAN_POINT('Origin',(-7.95655,4.3419873081547,-0.871973318823906));
#57634=CARTESIAN_POINT('',(7.95654999999997,7.8979873081547,-0.871973318823906));
#57635=CARTESIAN_POINT('',(-7.95654999999997,7.8979873081547,-0.871973318823906));
#57636=CARTESIAN_POINT('',(9.96068066769246,7.27943454458544,-0.871973318823906));
#57637=CARTESIAN_POINT('Origin',(7.95655,4.3419873081547,-0.871973318823906));
#57638=CARTESIAN_POINT('',(16.2281306676925,3.00334454458544,-0.871973318823906));
#57639=CARTESIAN_POINT('',(9.96068066769246,7.27943454458544,-0.871973318823906));
#57640=CARTESIAN_POINT('',(16.2281306676925,-2.87154992827604,-0.871973318823906));
#57641=CARTESIAN_POINT('Origin',(14.224,0.0658973081546998,-0.871973318823906));
#57642=CARTESIAN_POINT('',(9.96068066769245,-7.14763992827604,-0.871973318823906));
#57643=CARTESIAN_POINT('',(16.2281306676925,-2.87154992827604,-0.871973318823906));
#57644=CARTESIAN_POINT('',(7.95654999999997,-7.7661926918453,-0.871973318823906));
#57645=CARTESIAN_POINT('Origin',(7.95655,-4.2101926918453,-0.871973318823906));
#57646=CARTESIAN_POINT('',(-7.95654999999997,-7.7661926918453,-0.871973318823906));
#57647=CARTESIAN_POINT('',(7.95654999999997,-7.7661926918453,-0.871973318823906));
#57648=CARTESIAN_POINT('',(-9.96068066769245,-7.14763992827604,-0.871973318823906));
#57649=CARTESIAN_POINT('Origin',(-7.95655,-4.2101926918453,-0.871973318823906));
#57650=CARTESIAN_POINT('',(-16.2281306676925,-2.87154992827604,-0.871973318823906));
#57651=CARTESIAN_POINT('',(-6.66749999999998,6.7778473081547,-0.871973318823906));
#57652=CARTESIAN_POINT('',(6.66749999999998,6.7778473081547,-0.871973318823906));
#57653=CARTESIAN_POINT('',(-6.66749999999998,6.7778473081547,-0.871973318823906));
#57654=CARTESIAN_POINT('',(-9.3345,4.11084730815468,-0.871973318823906));
#57655=CARTESIAN_POINT('Origin',(-6.6675,4.1108473081547,-0.871973318823906));
#57656=CARTESIAN_POINT('',(-9.3345,-1.09634512099625,-0.871973318823906));
#57657=CARTESIAN_POINT('',(-9.3345,4.11084730815468,-0.871973318823906));
#57658=CARTESIAN_POINT('',(-8.55335378542452,-2.98219890642078,-0.871973318823906));
#57659=CARTESIAN_POINT('Origin',(-6.6675,-1.09634512099626,-0.871973318823906));
#57660=CARTESIAN_POINT('',(-5.67064621457553,-5.8649064772698,-0.871973318823906));
#57661=CARTESIAN_POINT('',(-8.55335378542452,-2.98219890642078,-0.871973318823906));
#57662=CARTESIAN_POINT('',(-3.78479242915098,-6.6460526918453,-0.871973318823906));
#57663=CARTESIAN_POINT('Origin',(-3.78479242915099,-3.9790526918453,-0.871973318823906));
#57664=CARTESIAN_POINT('',(3.784792429151,-6.6460526918453,-0.871973318823906));
#57665=CARTESIAN_POINT('',(3.784792429151,-6.6460526918453,-0.871973318823906));
#57666=CARTESIAN_POINT('',(5.67064621457553,-5.86490647726981,-0.871973318823906));
#57667=CARTESIAN_POINT('Origin',(3.78479242915099,-3.9790526918453,-0.871973318823906));
#57668=CARTESIAN_POINT('',(8.55335378542453,-2.98219890642078,-0.871973318823906));
#57669=CARTESIAN_POINT('',(8.55335378542453,-2.98219890642078,-0.871973318823906));
#57670=CARTESIAN_POINT('',(9.3345,-1.09634512099626,-0.871973318823906));
#57671=CARTESIAN_POINT('Origin',(6.6675,-1.09634512099626,-0.871973318823906));
#57672=CARTESIAN_POINT('',(9.3345,4.11084730815468,-0.871973318823906));
#57673=CARTESIAN_POINT('',(9.3345,-1.09634512099627,-0.871973318823906));
#57674=CARTESIAN_POINT('Origin',(6.6675,4.1108473081547,-0.871973318823906));
#57675=CARTESIAN_POINT('Origin',(-7.95655,4.3419873081547,3.37744668117609));
#57676=CARTESIAN_POINT('',(-11.51255,4.34198730815467,3.02184668117609));
#57677=CARTESIAN_POINT('',(-11.51255,4.34198730815467,1.33274668117609));
#57678=CARTESIAN_POINT('',(-11.51255,4.34198730815467,3.37744668117609));
#57679=CARTESIAN_POINT('',(-7.95654999999997,7.8979873081547,3.02184668117609));
#57680=CARTESIAN_POINT('Origin',(-7.95655,4.3419873081547,3.02184668117609));
#57681=CARTESIAN_POINT('',(-7.95654999999997,7.8979873081547,3.37744668117609));
#57682=CARTESIAN_POINT('',(-9.96068066769246,7.27943454458544,1.33274668117609));
#57683=CARTESIAN_POINT('',(-9.96068066769246,7.27943454458544,1.33274668117609));
#57684=CARTESIAN_POINT('Origin',(-7.95655,4.3419873081547,1.33274668117609));
#57685=CARTESIAN_POINT('Origin',(-11.51255,4.34198730815467,3.37744668117609));
#57686=CARTESIAN_POINT('',(-11.51255,-4.21019269184527,3.02184668117609));
#57687=CARTESIAN_POINT('',(-11.51255,-4.21019269184527,1.33274668117609));
#57688=CARTESIAN_POINT('',(-11.51255,-4.21019269184527,3.37744668117609));
#57689=CARTESIAN_POINT('',(-11.51255,4.34198730815467,3.02184668117609));
#57690=CARTESIAN_POINT('',(-11.51255,4.34198730815467,1.33274668117609));
#57691=CARTESIAN_POINT('Origin',(7.95655,-4.2101926918453,3.37744668117609));
#57692=CARTESIAN_POINT('',(11.51255,-4.21019269184527,3.02184668117609));
#57693=CARTESIAN_POINT('',(11.51255,-4.21019269184527,1.33274668117609));
#57694=CARTESIAN_POINT('',(11.51255,-4.21019269184527,3.37744668117609));
#57695=CARTESIAN_POINT('',(7.95654999999997,-7.7661926918453,3.02184668117609));
#57696=CARTESIAN_POINT('Origin',(7.95655,-4.2101926918453,3.02184668117609));
#57697=CARTESIAN_POINT('',(7.95654999999997,-7.7661926918453,3.37744668117609));
#57698=CARTESIAN_POINT('',(9.96068066769245,-7.14763992827604,1.33274668117609));
#57699=CARTESIAN_POINT('',(9.96068066769245,-7.14763992827604,1.33274668117609));
#57700=CARTESIAN_POINT('Origin',(7.95655,-4.2101926918453,1.33274668117609));
#57701=CARTESIAN_POINT('Origin',(11.51255,-4.21019269184527,3.37744668117609));
#57702=CARTESIAN_POINT('',(11.51255,4.34198730815467,3.02184668117609));
#57703=CARTESIAN_POINT('',(11.51255,4.34198730815467,1.33274668117609));
#57704=CARTESIAN_POINT('',(11.51255,4.34198730815467,3.37744668117609));
#57705=CARTESIAN_POINT('',(11.51255,-4.21019269184527,3.02184668117609));
#57706=CARTESIAN_POINT('',(11.51255,-4.21019269184527,1.33274668117609));
#57707=CARTESIAN_POINT('Origin',(7.95655,4.3419873081547,3.37744668117609));
#57708=CARTESIAN_POINT('',(7.95654999999997,7.8979873081547,3.02184668117609));
#57709=CARTESIAN_POINT('',(7.95654999999997,7.8979873081547,3.37744668117609));
#57710=CARTESIAN_POINT('Origin',(7.95655,4.3419873081547,3.02184668117609));
#57711=CARTESIAN_POINT('',(9.96068066769246,7.27943454458544,1.33274668117609));
#57712=CARTESIAN_POINT('Origin',(7.95655,4.3419873081547,1.33274668117609));
#57713=CARTESIAN_POINT('',(9.96068066769246,7.27943454458544,1.33274668117609));
#57714=CARTESIAN_POINT('Origin',(-7.95654999999997,7.8979873081547,3.37744668117609));
#57715=CARTESIAN_POINT('',(7.95654999999997,7.8979873081547,3.02184668117609));
#57716=CARTESIAN_POINT('Origin',(-7.95655,-4.2101926918453,3.37744668117609));
#57717=CARTESIAN_POINT('',(-7.95654999999997,-7.7661926918453,3.02184668117609));
#57718=CARTESIAN_POINT('',(-7.95654999999997,-7.7661926918453,3.37744668117609));
#57719=CARTESIAN_POINT('Origin',(-7.95655,-4.2101926918453,3.02184668117609));
#57720=CARTESIAN_POINT('',(-9.96068066769245,-7.14763992827604,1.33274668117609));
#57721=CARTESIAN_POINT('Origin',(-7.95655,-4.2101926918453,1.33274668117609));
#57722=CARTESIAN_POINT('',(-9.96068066769245,-7.14763992827604,1.33274668117609));
#57723=CARTESIAN_POINT('Origin',(7.95654999999997,-7.7661926918453,3.37744668117609));
#57724=CARTESIAN_POINT('',(-7.95654999999997,-7.7661926918453,3.02184668117609));
#57725=CARTESIAN_POINT('Origin',(16.2281306676925,-2.87154992827604,1.33274668117609));
#57726=CARTESIAN_POINT('',(16.2281306676925,-2.87154992827604,1.33274668117609));
#57727=CARTESIAN_POINT('',(16.2281306676925,-2.87154992827604,1.33274668117609));
#57728=CARTESIAN_POINT('',(16.2281306676925,-2.87154992827604,1.33274668117609));
#57729=CARTESIAN_POINT('Origin',(14.224,0.0658973081546998,1.33274668117609));
#57730=CARTESIAN_POINT('',(16.2281306676925,3.00334454458544,1.33274668117609));
#57731=CARTESIAN_POINT('',(16.2281306676925,3.00334454458544,1.33274668117609));
#57732=CARTESIAN_POINT('Origin',(14.224,0.0658973081546998,1.33274668117609));
#57733=CARTESIAN_POINT('Origin',(9.96068066769246,7.27943454458544,1.33274668117609));
#57734=CARTESIAN_POINT('',(9.96068066769246,7.27943454458544,1.33274668117609));
#57735=CARTESIAN_POINT('Origin',(7.95655,4.3419873081547,1.33274668117609));
#57736=CARTESIAN_POINT('Origin',(-9.96068066769246,7.27943454458544,1.33274668117609));
#57737=CARTESIAN_POINT('',(-9.96068066769246,7.27943454458544,1.33274668117609));
#57738=CARTESIAN_POINT('Origin',(-16.2281306676925,-2.87154992827604,1.33274668117609));
#57739=CARTESIAN_POINT('',(-16.2281306676925,-2.87154992827604,1.33274668117609));
#57740=CARTESIAN_POINT('Origin',(-7.95655,4.3419873081547,1.33274668117609));
#57741=CARTESIAN_POINT('Origin',(7.95655,4.3419873081547,3.02184668117609));
#57742=CARTESIAN_POINT('Origin',(7.95654999999997,7.5423873081547,3.02184668117609));
#57743=CARTESIAN_POINT('Origin',(11.15695,4.34198730815468,3.02184668117609));
#57744=CARTESIAN_POINT('Origin',(11.15695,-4.2101926918453,3.02184668117609));
#57745=CARTESIAN_POINT('Origin',(11.15695,-4.21019269184527,3.02184668117609));
#57746=CARTESIAN_POINT('Origin',(-7.95654999999997,7.5423873081547,3.02184668117609));
#57747=CARTESIAN_POINT('Origin',(-7.95654999999997,7.5423873081547,3.02184668117609));
#57748=CARTESIAN_POINT('Origin',(7.95655,-4.2101926918453,3.02184668117609));
#57749=CARTESIAN_POINT('Origin',(7.95654999999997,-7.4105926918453,3.02184668117609));
#57750=CARTESIAN_POINT('Origin',(-7.95655,4.3419873081547,3.02184668117609));
#57751=CARTESIAN_POINT('Origin',(-11.15695,4.34198730815467,3.02184668117609));
#57752=CARTESIAN_POINT('Origin',(7.95654999999997,-7.4105926918453,3.02184668117609));
#57753=CARTESIAN_POINT('Origin',(-7.95654999999997,-7.4105926918453,3.02184668117609));
#57754=CARTESIAN_POINT('Origin',(-11.15695,-4.2101926918453,3.02184668117609));
#57755=CARTESIAN_POINT('Origin',(-11.15695,-4.21019269184528,3.02184668117609));
#57756=CARTESIAN_POINT('Origin',(-7.95655,-4.2101926918453,3.02184668117609));
#57757=CARTESIAN_POINT('Origin',(-6.6675,4.1108473081547,-10.0286733188239));
#57758=CARTESIAN_POINT('',(-6.66749999999998,6.7778473081547,-10.0286733188239));
#57759=CARTESIAN_POINT('',(-9.3345,4.11084730815468,-10.0286733188239));
#57760=CARTESIAN_POINT('Origin',(-6.66749999999998,6.7778473081547,-10.0286733188239));
#57761=CARTESIAN_POINT('',(6.66749999999998,6.7778473081547,-10.0286733188239));
#57762=CARTESIAN_POINT('Origin',(6.6675,4.1108473081547,-10.0286733188239));
#57763=CARTESIAN_POINT('',(9.3345,4.11084730815468,-10.0286733188239));
#57764=CARTESIAN_POINT('Origin',(9.3345,-1.09634512099627,-10.0286733188239));
#57765=CARTESIAN_POINT('',(9.3345,-1.09634512099626,-10.0286733188239));
#57766=CARTESIAN_POINT('Origin',(6.6675,-1.09634512099626,-10.0286733188239));
#57767=CARTESIAN_POINT('',(8.55335378542453,-2.98219890642078,-10.0286733188239));
#57768=CARTESIAN_POINT('Origin',(8.55335378542453,-2.98219890642078,-10.0286733188239));
#57769=CARTESIAN_POINT('',(5.67064621457553,-5.86490647726981,-10.0286733188239));
#57770=CARTESIAN_POINT('Origin',(3.78479242915099,-3.9790526918453,-10.0286733188239));
#57771=CARTESIAN_POINT('',(3.784792429151,-6.6460526918453,-10.0286733188239));
#57772=CARTESIAN_POINT('Origin',(3.784792429151,-6.6460526918453,-10.0286733188239));
#57773=CARTESIAN_POINT('',(-3.78479242915098,-6.6460526918453,-10.0286733188239));
#57774=CARTESIAN_POINT('Origin',(-3.78479242915099,-3.9790526918453,-10.0286733188239));
#57775=CARTESIAN_POINT('',(-5.67064621457553,-5.8649064772698,-10.0286733188239));
#57776=CARTESIAN_POINT('Origin',(-8.55335378542452,-2.98219890642078,-10.0286733188239));
#57777=CARTESIAN_POINT('',(-8.55335378542452,-2.98219890642078,-10.0286733188239));
#57778=CARTESIAN_POINT('Origin',(-6.6675,-1.09634512099626,-10.0286733188239));
#57779=CARTESIAN_POINT('',(-9.3345,-1.09634512099625,-10.0286733188239));
#57780=CARTESIAN_POINT('Origin',(-9.3345,4.11084730815468,-10.0286733188239));
#57781=CARTESIAN_POINT('Origin',(-4.15302828610066,-3.7123526918453,-8.42847331882391));
#57782=CARTESIAN_POINT('',(-4.15302828610065,-5.4903526918453,-8.42847331882391));
#57783=CARTESIAN_POINT('',(-5.41026414305035,-4.96958854879497,-8.42847331882391));
#57784=CARTESIAN_POINT('Origin',(-7.92473585694968,-2.45511683489562,-8.42847331882391));
#57785=CARTESIAN_POINT('',(-7.92473585694968,-2.45511683489562,-8.42847331882391));
#57786=CARTESIAN_POINT('Origin',(-6.6675,-1.19788097794594,-8.42847331882391));
#57787=CARTESIAN_POINT('',(-8.4455,-1.19788097794593,-8.42847331882391));
#57788=CARTESIAN_POINT('Origin',(-8.4455,3.84414730815469,-8.42847331882391));
#57789=CARTESIAN_POINT('',(-8.4455,3.84414730815469,-8.42847331882391));
#57790=CARTESIAN_POINT('Origin',(-6.6675,3.8441473081547,-8.42847331882391));
#57791=CARTESIAN_POINT('',(-6.66749999999999,5.6221473081547,-8.42847331882391));
#57792=CARTESIAN_POINT('Origin',(-6.66749999999999,5.6221473081547,-8.42847331882391));
#57793=CARTESIAN_POINT('',(6.66749999999999,5.6221473081547,-8.42847331882391));
#57794=CARTESIAN_POINT('Origin',(6.6675,3.8441473081547,-8.42847331882391));
#57795=CARTESIAN_POINT('',(8.4455,3.84414730815469,-8.42847331882391));
#57796=CARTESIAN_POINT('Origin',(8.4455,-1.19788097794593,-8.42847331882391));
#57797=CARTESIAN_POINT('',(8.4455,-1.19788097794593,-8.42847331882391));
#57798=CARTESIAN_POINT('Origin',(6.6675,-1.19788097794594,-8.42847331882391));
#57799=CARTESIAN_POINT('',(7.92473585694968,-2.45511683489562,-8.42847331882391));
#57800=CARTESIAN_POINT('Origin',(7.92473585694968,-2.45511683489562,-8.42847331882391));
#57801=CARTESIAN_POINT('',(5.41026414305036,-4.96958854879497,-8.42847331882391));
#57802=CARTESIAN_POINT('Origin',(4.15302828610066,-3.7123526918453,-8.42847331882391));
#57803=CARTESIAN_POINT('',(4.15302828610066,-5.4903526918453,-8.42847331882391));
#57804=CARTESIAN_POINT('Origin',(4.15302828610066,-5.4903526918453,-8.42847331882391));
#57805=CARTESIAN_POINT('Origin',(0.70231,-3.0900526918453,0.194826681176092));
#57806=CARTESIAN_POINT('',(0.70231,-3.0900526918453,2.11901678258961));
#57807=CARTESIAN_POINT('Origin',(-3.92938,0.2881473081547,0.194826681176092));
#57808=CARTESIAN_POINT('',(-3.92938,0.288147308154702,-1.2256693468728));
#57809=CARTESIAN_POINT('Origin',(5.334,3.2218473081547,0.194826681176092));
#57810=CARTESIAN_POINT('',(5.334,3.2218473081547,-1.2256693468728));
#57811=CARTESIAN_POINT('Origin',(-4.36283493912025,9.41566770809984,0.729519532971223));
#57812=CARTESIAN_POINT('Origin',(-4.90054506087975,9.41566770809984,0.729519532971223));
#57813=CARTESIAN_POINT('Origin',(4.90054506087975,9.41566770809984,0.729519532971222));
#57814=CARTESIAN_POINT('Origin',(4.36283493912025,9.41566770809984,0.729519532971222));
#57815=CARTESIAN_POINT('Origin',(-0.2667,3.97571428641218,3.37744668117609));
#57816=CARTESIAN_POINT('Origin',(0.2667,3.97571428641218,3.37744668117609));
#57817=CARTESIAN_POINT('Origin',(1.41351,0.554847308154699,-11.0954733188239));
#57818=CARTESIAN_POINT('',(-1.41351,0.554847308154699,-11.0954733188239));
#57819=CARTESIAN_POINT('',(1.41351,0.554847308154699,-11.0954733188239));
#57820=CARTESIAN_POINT('',(-1.41351,0.554847308154699,-11.0954733188239));
#57821=CARTESIAN_POINT('',(1.41351,-3.8012526918453,-11.0954733188239));
#57822=CARTESIAN_POINT('',(1.41351,-3.8012526918453,-11.0954733188239));
#57823=CARTESIAN_POINT('',(-1.41351,-3.8012526918453,-11.0954733188239));
#57824=CARTESIAN_POINT('',(1.41351,-3.8012526918453,-11.0954733188239));
#57825=CARTESIAN_POINT('',(-1.41351,0.554847308154699,-11.0954733188239));
#57826=CARTESIAN_POINT('',(0.451338313394325,-0.156352691845301,-11.0954733188239));
#57827=CARTESIAN_POINT('',(-0.451338313394325,-0.156352691845301,-11.0954733188239));
#57828=CARTESIAN_POINT('',(-0.451338313394325,-0.156352691845301,-11.0954733188239));
#57829=CARTESIAN_POINT('',(-0.451338313394325,-3.0900526918453,-11.0954733188239));
#57830=CARTESIAN_POINT('',(-0.451338313394325,-3.0900526918453,-11.0954733188239));
#57831=CARTESIAN_POINT('',(0.451338313394325,-3.0900526918453,-11.0954733188239));
#57832=CARTESIAN_POINT('',(0.451338313394325,-3.0900526918453,-11.0954733188239));
#57833=CARTESIAN_POINT('',(0.451338313394325,-3.0900526918453,-11.0954733188239));
#57834=CARTESIAN_POINT('Origin',(-1.41351,0.554847308154699,-11.0954733188239));
#57835=CARTESIAN_POINT('',(1.41351,0.554847308154699,-11.0954733188239));
#57836=CARTESIAN_POINT('',(-1.41351,0.554847308154699,-11.0954733188239));
#57837=CARTESIAN_POINT('Origin',(1.41351,-3.8012526918453,-11.0954733188239));
#57838=CARTESIAN_POINT('',(1.41351,-3.8012526918453,-11.0954733188239));
#57839=CARTESIAN_POINT('Origin',(1.41351,-3.8012526918453,-11.0954733188239));
#57840=CARTESIAN_POINT('',(-1.41351,-3.8012526918453,-11.0954733188239));
#57841=CARTESIAN_POINT('Origin',(-1.41351,0.554847308154699,-11.0954733188239));
#57842=CARTESIAN_POINT('Origin',(-17.78,-1.6232026918453,-16.8055370922563));
#57843=CARTESIAN_POINT('',(-0.451338313394325,-1.06933891841287,-16.2516733188239));
#57844=CARTESIAN_POINT('',(-0.451338313394325,-0.156352691845301,-15.3386870922563));
#57845=CARTESIAN_POINT('',(-0.451338313394325,-2.07969580512908,-17.2620302055401));
#57846=CARTESIAN_POINT('',(0.451338313394325,-0.156352691845301,-15.3386870922563));
#57847=CARTESIAN_POINT('',(-0.451338313394325,-0.156352691845301,-15.3386870922563));
#57848=CARTESIAN_POINT('',(0.451338313394325,-1.06933891841287,-16.2516733188239));
#57849=CARTESIAN_POINT('',(0.451338313394325,-2.07969580512908,-17.2620302055401));
#57850=CARTESIAN_POINT('',(-0.451338313394325,-1.06933891841287,-16.2516733188239));
#57851=CARTESIAN_POINT('Origin',(-0.451338313394325,-3.0900526918453,-16.2516733188239));
#57852=CARTESIAN_POINT('',(0.451338313394325,-2.17706646527773,-16.2516733188239));
#57853=CARTESIAN_POINT('',(0.451338313394325,-3.0900526918453,-16.2516733188239));
#57854=CARTESIAN_POINT('',(-0.451338313394325,-2.17706646527773,-16.2516733188239));
#57855=CARTESIAN_POINT('',(-0.451338313394325,-2.17706646527773,-16.2516733188239));
#57856=CARTESIAN_POINT('',(-0.451338313394325,-3.0900526918453,-16.2516733188239));
#57857=CARTESIAN_POINT('Origin',(-17.78,-1.6232026918453,-16.8055370922563));
#57858=CARTESIAN_POINT('',(-0.451338313394325,-3.0900526918453,-15.3386870922563));
#57859=CARTESIAN_POINT('',(-0.451338313394325,-2.63355957856152,-15.7951802055401));
#57860=CARTESIAN_POINT('',(0.451338313394325,-3.0900526918453,-15.3386870922563));
#57861=CARTESIAN_POINT('',(0.451338313394325,-2.63355957856152,-15.7951802055401));
#57862=CARTESIAN_POINT('',(0.451338313394325,-3.0900526918453,-15.3386870922563));
#57863=CARTESIAN_POINT('Origin',(0.451338313394325,-3.0900526918453,-16.2516733188239));
#57864=CARTESIAN_POINT('',(-0.451338313394325,-3.0900526918453,-16.2516733188239));
#57865=CARTESIAN_POINT('',(0.451338313394325,-3.0900526918453,-16.2516733188239));
#57866=CARTESIAN_POINT('Origin',(0.451338313394325,-3.0900526918453,-16.2516733188239));
#57867=CARTESIAN_POINT('',(0.451338313394325,-0.156352691845301,-16.2516733188239));
#57868=CARTESIAN_POINT('Origin',(-0.451338313394325,-0.156352691845301,
-16.2516733188239));
#57869=CARTESIAN_POINT('',(-0.451338313394325,-0.156352691845301,-16.2516733188239));
#57870=CARTESIAN_POINT('Origin',(-0.451338313394325,-3.0900526918453,-16.2516733188239));
#57871=CARTESIAN_POINT('Origin',(3.21818,-0.4230526918453,-11.0954733188239));
#57872=CARTESIAN_POINT('',(3.21818,-0.4230526918453,-11.0954733188239));
#57873=CARTESIAN_POINT('',(3.21818,-0.4230526918453,-11.0954733188239));
#57874=CARTESIAN_POINT('',(6.0452,-0.4230526918453,-11.0954733188239));
#57875=CARTESIAN_POINT('',(3.21818,-0.4230526918453,-11.0954733188239));
#57876=CARTESIAN_POINT('',(6.0452,-0.4230526918453,-11.0954733188239));
#57877=CARTESIAN_POINT('Origin',(3.21818,-0.4230526918453,-11.0954733188239));
#57878=CARTESIAN_POINT('',(3.21818,3.9330473081547,-11.0954733188239));
#57879=CARTESIAN_POINT('',(3.21818,3.9330473081547,-11.0954733188239));
#57880=CARTESIAN_POINT('',(3.21818,-0.4230526918453,-11.0954733188239));
#57881=CARTESIAN_POINT('Origin',(6.0452,3.9330473081547,-11.0954733188239));
#57882=CARTESIAN_POINT('',(6.0452,3.9330473081547,-11.0954733188239));
#57883=CARTESIAN_POINT('',(6.0452,3.9330473081547,-11.0954733188239));
#57884=CARTESIAN_POINT('',(6.0452,3.9330473081547,-11.0954733188239));
#57885=CARTESIAN_POINT('Origin',(6.0452,3.9330473081547,-11.0954733188239));
#57886=CARTESIAN_POINT('',(6.0452,3.9330473081547,-11.0954733188239));
#57887=CARTESIAN_POINT('Origin',(6.0452,-0.423052691845299,-11.0954733188239));
#57888=CARTESIAN_POINT('',(5.01908361227606,3.2218473081547,-11.0954733188239));
#57889=CARTESIAN_POINT('',(5.01908361227606,0.2881473081547,-11.0954733188239));
#57890=CARTESIAN_POINT('',(5.01908361227606,3.2218473081547,-11.0954733188239));
#57891=CARTESIAN_POINT('',(4.24429638772394,3.2218473081547,-11.0954733188239));
#57892=CARTESIAN_POINT('',(5.01908361227606,3.2218473081547,-11.0954733188239));
#57893=CARTESIAN_POINT('',(4.24429638772394,0.2881473081547,-11.0954733188239));
#57894=CARTESIAN_POINT('',(4.24429638772394,3.2218473081547,-11.0954733188239));
#57895=CARTESIAN_POINT('',(4.24429638772394,0.2881473081547,-11.0954733188239));
#57896=CARTESIAN_POINT('Origin',(5.01908361227606,0.2881473081547,-16.2516733188239));
#57897=CARTESIAN_POINT('',(5.01908361227606,2.30886108158713,-16.2516733188239));
#57898=CARTESIAN_POINT('',(5.01908361227606,1.20113353472227,-16.2516733188239));
#57899=CARTESIAN_POINT('',(5.01908361227606,3.2218473081547,-16.2516733188239));
#57900=CARTESIAN_POINT('',(4.24429638772394,1.20113353472227,-16.2516733188239));
#57901=CARTESIAN_POINT('',(5.01908361227606,1.20113353472227,-16.2516733188239));
#57902=CARTESIAN_POINT('',(4.24429638772394,2.30886108158713,-16.2516733188239));
#57903=CARTESIAN_POINT('',(4.24429638772394,3.2218473081547,-16.2516733188239));
#57904=CARTESIAN_POINT('',(5.01908361227606,2.30886108158713,-16.2516733188239));
#57905=CARTESIAN_POINT('Origin',(-17.78,1.7549973081547,-16.8055370922563));
#57906=CARTESIAN_POINT('',(5.01908361227606,3.2218473081547,-15.3386870922563));
#57907=CARTESIAN_POINT('',(5.01908361227606,1.7549973081547,-16.8055370922563));
#57908=CARTESIAN_POINT('',(4.24429638772394,3.2218473081547,-15.3386870922563));
#57909=CARTESIAN_POINT('',(4.24429638772394,2.76535419487092,-15.7951802055401));
#57910=CARTESIAN_POINT('',(5.01908361227606,3.2218473081547,-15.3386870922563));
#57911=CARTESIAN_POINT('Origin',(-17.78,1.7549973081547,-16.8055370922563));
#57912=CARTESIAN_POINT('',(5.01908361227606,0.2881473081547,-15.3386870922563));
#57913=CARTESIAN_POINT('',(4.24429638772394,0.2881473081547,-15.3386870922563));
#57914=CARTESIAN_POINT('',(4.24429638772394,0.2881473081547,-15.3386870922563));
#57915=CARTESIAN_POINT('',(4.24429638772394,2.21149042143848,-17.2620302055401));
#57916=CARTESIAN_POINT('',(5.01908361227606,1.7549973081547,-16.8055370922563));
#57917=CARTESIAN_POINT('Origin',(4.24429638772394,0.2881473081547,-16.2516733188239));
#57918=CARTESIAN_POINT('',(4.24429638772394,0.2881473081547,-16.2516733188239));
#57919=CARTESIAN_POINT('',(5.01908361227606,0.2881473081547,-16.2516733188239));
#57920=CARTESIAN_POINT('Origin',(5.01908361227606,3.2218473081547,-16.2516733188239));
#57921=CARTESIAN_POINT('',(5.01908361227606,3.2218473081547,-16.2516733188239));
#57922=CARTESIAN_POINT('',(4.24429638772394,3.2218473081547,-16.2516733188239));
#57923=CARTESIAN_POINT('Origin',(4.24429638772394,3.2218473081547,-16.2516733188239));
#57924=CARTESIAN_POINT('Origin',(5.01908361227606,3.2218473081547,-16.2516733188239));
#57925=CARTESIAN_POINT('Origin',(-3.21818,-0.4230526918453,-11.0954733188239));
#57926=CARTESIAN_POINT('',(-3.21818,-0.4230526918453,-11.0954733188239));
#57927=CARTESIAN_POINT('',(-3.21818,3.9330473081547,-11.0954733188239));
#57928=CARTESIAN_POINT('',(-3.21818,-0.4230526918453,-11.0954733188239));
#57929=CARTESIAN_POINT('',(-6.0452,-0.4230526918453,-11.0954733188239));
#57930=CARTESIAN_POINT('',(-3.21818,-0.4230526918453,-11.0954733188239));
#57931=CARTESIAN_POINT('',(-6.0452,3.9330473081547,-11.0954733188239));
#57932=CARTESIAN_POINT('',(-6.0452,3.9330473081547,-11.0954733188239));
#57933=CARTESIAN_POINT('',(-6.0452,3.9330473081547,-11.0954733188239));
#57934=CARTESIAN_POINT('',(-4.24429638772394,3.2218473081547,-11.0954733188239));
#57935=CARTESIAN_POINT('',(-4.24429638772394,0.2881473081547,-11.0954733188239));
#57936=CARTESIAN_POINT('',(-4.24429638772394,0.2881473081547,-11.0954733188239));
#57937=CARTESIAN_POINT('',(-5.01908361227606,3.2218473081547,-11.0954733188239));
#57938=CARTESIAN_POINT('',(-5.01908361227606,3.2218473081547,-11.0954733188239));
#57939=CARTESIAN_POINT('',(-5.01908361227606,0.2881473081547,-11.0954733188239));
#57940=CARTESIAN_POINT('',(-5.01908361227606,0.2881473081547,-11.0954733188239));
#57941=CARTESIAN_POINT('',(-4.24429638772394,0.2881473081547,-11.0954733188239));
#57942=CARTESIAN_POINT('Origin',(-3.21818,-0.4230526918453,-11.0954733188239));
#57943=CARTESIAN_POINT('',(-3.21818,-0.4230526918453,-11.0954733188239));
#57944=CARTESIAN_POINT('',(-3.21818,3.9330473081547,-11.0954733188239));
#57945=CARTESIAN_POINT('Origin',(-3.21818,-0.4230526918453,-11.0954733188239));
#57946=CARTESIAN_POINT('',(-6.0452,-0.4230526918453,-11.0954733188239));
#57947=CARTESIAN_POINT('Origin',(-6.0452,3.9330473081547,-11.0954733188239));
#57948=CARTESIAN_POINT('',(-6.0452,3.9330473081547,-11.0954733188239));
#57949=CARTESIAN_POINT('Origin',(-6.0452,3.9330473081547,-11.0954733188239));
#57950=CARTESIAN_POINT('Origin',(-4.24429638772394,3.2218473081547,-16.2516733188239));
#57951=CARTESIAN_POINT('',(-5.01908361227606,1.20113353472227,-16.2516733188239));
#57952=CARTESIAN_POINT('',(-4.24429638772394,1.20113353472227,-16.2516733188239));
#57953=CARTESIAN_POINT('',(-4.24429638772394,1.20113353472227,-16.2516733188239));
#57954=CARTESIAN_POINT('',(-5.01908361227606,2.30886108158713,-16.2516733188239));
#57955=CARTESIAN_POINT('',(-5.01908361227606,0.2881473081547,-16.2516733188239));
#57956=CARTESIAN_POINT('',(-4.24429638772394,2.30886108158713,-16.2516733188239));
#57957=CARTESIAN_POINT('',(-4.24429638772394,2.30886108158713,-16.2516733188239));
#57958=CARTESIAN_POINT('',(-4.24429638772394,0.2881473081547,-16.2516733188239));
#57959=CARTESIAN_POINT('Origin',(-17.78,1.7549973081547,-16.8055370922563));
#57960=CARTESIAN_POINT('',(-5.01908361227606,3.2218473081547,-15.3386870922563));
#57961=CARTESIAN_POINT('',(-4.24429638772394,3.2218473081547,-15.3386870922563));
#57962=CARTESIAN_POINT('',(-5.01908361227606,3.2218473081547,-15.3386870922563));
#57963=CARTESIAN_POINT('',(-4.24429638772394,1.29850419487091,-17.2620302055401));
#57964=CARTESIAN_POINT('',(-5.01908361227606,1.29850419487091,-17.2620302055401));
#57965=CARTESIAN_POINT('Origin',(-17.78,1.7549973081547,-16.8055370922563));
#57966=CARTESIAN_POINT('',(-4.24429638772394,0.2881473081547,-15.3386870922563));
#57967=CARTESIAN_POINT('',(-4.24429638772394,0.744640421438487,-15.7951802055401));
#57968=CARTESIAN_POINT('',(-5.01908361227606,0.2881473081547,-15.3386870922563));
#57969=CARTESIAN_POINT('',(-4.24429638772394,0.2881473081547,-15.3386870922563));
#57970=CARTESIAN_POINT('',(-5.01908361227606,0.744640421438487,-15.7951802055401));
#57971=CARTESIAN_POINT('Origin',(-4.24429638772394,0.2881473081547,-16.2516733188239));
#57972=CARTESIAN_POINT('',(-5.01908361227606,0.2881473081547,-16.2516733188239));
#57973=CARTESIAN_POINT('',(-4.24429638772394,0.2881473081547,-16.2516733188239));
#57974=CARTESIAN_POINT('Origin',(-5.01908361227606,3.2218473081547,-16.2516733188239));
#57975=CARTESIAN_POINT('',(-4.24429638772394,3.2218473081547,-16.2516733188239));
#57976=CARTESIAN_POINT('',(-5.01908361227606,3.2218473081547,-16.2516733188239));
#57977=CARTESIAN_POINT('Origin',(-5.01908361227606,0.2881473081547,-16.2516733188239));
#57978=CARTESIAN_POINT('Origin',(-4.24429638772394,0.2881473081547,-16.2516733188239));
#65295=UNCERTAINTY_MEASURE_WITH_UNIT(LENGTH_MEASURE(0.01),#65305,
'DISTANCE_ACCURACY_VALUE',
'Maximum model space distance between geometric entities at asserted c
onnectivities');
#65298=UNCERTAINTY_MEASURE_WITH_UNIT(LENGTH_MEASURE(0.01),#65305,
'DISTANCE_ACCURACY_VALUE',
'Maximum model space distance between geometric entities at asserted c
onnectivities');
#65301=(
GEOMETRIC_REPRESENTATION_CONTEXT(3)
GLOBAL_UNCERTAINTY_ASSIGNED_CONTEXT((#65295))
GLOBAL_UNIT_ASSIGNED_CONTEXT((#65305,#65307,#65308))
REPRESENTATION_CONTEXT('','3D')
);
#65304=(
GEOMETRIC_REPRESENTATION_CONTEXT(3)
GLOBAL_UNCERTAINTY_ASSIGNED_CONTEXT((#65298))
GLOBAL_UNIT_ASSIGNED_CONTEXT((#65305,#65307,#65308))
REPRESENTATION_CONTEXT('','3D')
);
#65305=(
LENGTH_UNIT()
NAMED_UNIT(*)
SI_UNIT(.MILLI.,.METRE.)
);
#65307=(
NAMED_UNIT(*)
PLANE_ANGLE_UNIT()
SI_UNIT($,.RADIAN.)
);
#65308=(
NAMED_UNIT(*)
SI_UNIT($,.STERADIAN.)
SOLID_ANGLE_UNIT()
);
#65311=SHAPE_DEFINITION_REPRESENTATION(#65316,#65325);
#65316=PRODUCT_DEFINITION_SHAPE('',$,#65331);
#65325=SHAPE_REPRESENTATION('',(#41041),#65301);
#65328=PRODUCT_DEFINITION_CONTEXT('part definition',#65345,'design');
#65331=PRODUCT_DEFINITION('AC Connector','AC Connector',#65336,#65328);
#65336=PRODUCT_DEFINITION_FORMATION('',$,#65349);
#65345=APPLICATION_CONTEXT(
'Core Data for Automotive Mechanical Design Process');
#65346=PRODUCT_CONTEXT('part definition',#65345,'mechanical');
#65349=PRODUCT('AC Connector','AC Connector',$,(#65346));
#65354=PRESENTATION_STYLE_ASSIGNMENT((#65359));
#65359=SURFACE_STYLE_USAGE(.BOTH.,#65364);
#65364=SURFACE_SIDE_STYLE('',(#65369));
#65369=SURFACE_STYLE_FILL_AREA(#65374);
#65374=FILL_AREA_STYLE('Opaque(23,69,131)',(#65379));
#65379=FILL_AREA_STYLE_COLOUR('Opaque(23,69,131)',#65384);
#65384=COLOUR_RGB('Opaque(23,69,131)',0.0901960784313725,0.270588235294118,
0.513725490196078);
ENDSEC;
END-ISO-10303-21;
